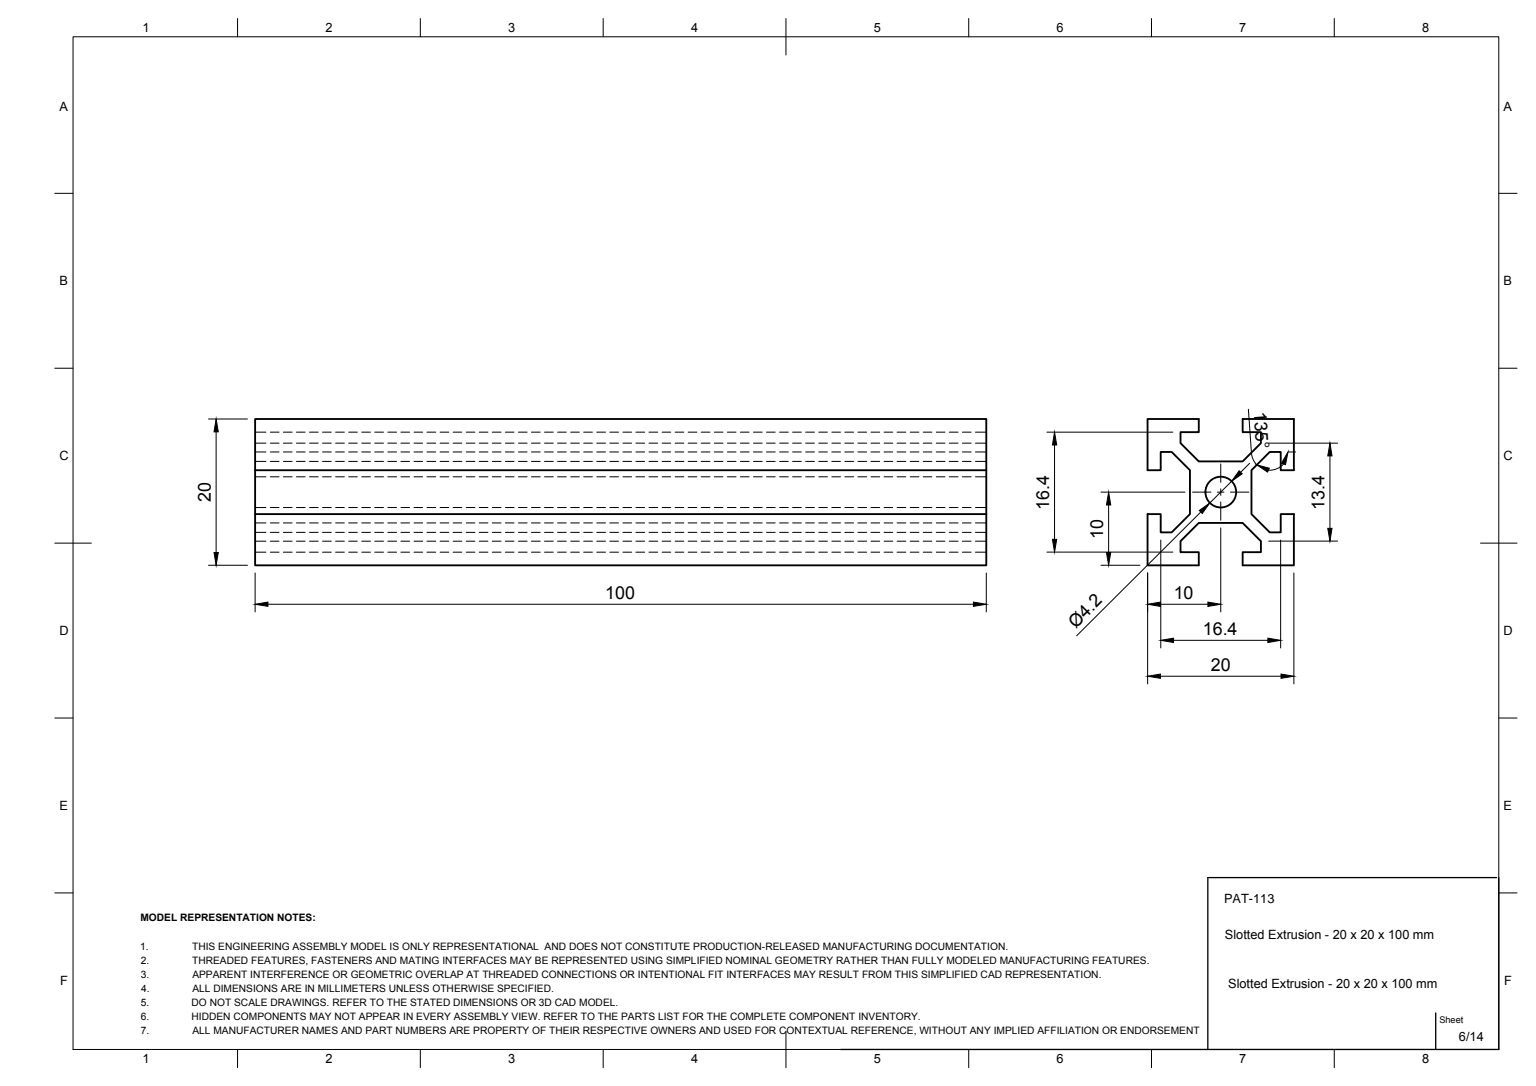
ISO-10303-21;
HEADER;
/* Generated by software containing ST-Developer
 * from STEP Tools, Inc. (www.steptools.com) 
 */

FILE_DESCRIPTION(
/* description */ ('Two-link friction support arm'),
/* implementation_level */ '2;1');

FILE_NAME(
/* name */ 'Slotted Extrusion - 20 x 20 x 100 mm.step',
/* time_stamp */ '2026-10-27T20:01:49-07:00',
/* author */ (''),
/* organization */ (''),
/* preprocessor_version */ 'ST-DEVELOPER v20.2',
/* originating_system */ 'Autodesk Translation Framework v15.17.0.0',
/* authorisation */ '');

FILE_SCHEMA (('AUTOMOTIVE_DESIGN { 1 0 10303 214 3 1 1 }'));
ENDSEC;

DATA;
#10=MECHANICAL_DESIGN_GEOMETRIC_PRESENTATION_REPRESENTATION('',(#196),#5492);
#174=SHAPE_REPRESENTATION_RELATIONSHIP('SRR','None',#5565,#185);
#185=ADVANCED_BREP_SHAPE_REPRESENTATION('',(#207),#5479);
#196=STYLED_ITEM('',(#5715),#207);
#207=MANIFOLD_SOLID_BREP('Body1',#3172);
#222=FACE_BOUND('',#605,.T.);
#223=FACE_BOUND('',#607,.T.);
#260=PLANE('',#3328);
#261=PLANE('',#3329);
#262=PLANE('',#3330);
#263=PLANE('',#3331);
#264=PLANE('',#3332);
#265=PLANE('',#3333);
#266=PLANE('',#3334);
#267=PLANE('',#3335);
#268=PLANE('',#3336);
#269=PLANE('',#3337);
#270=PLANE('',#3338);
#271=PLANE('',#3339);
#272=PLANE('',#3340);
#273=PLANE('',#3341);
#274=PLANE('',#3342);
#275=PLANE('',#3343);
#276=PLANE('',#3344);
#277=PLANE('',#3345);
#278=PLANE('',#3346);
#279=PLANE('',#3347);
#280=PLANE('',#3348);
#281=PLANE('',#3349);
#282=PLANE('',#3350);
#283=PLANE('',#3351);
#284=PLANE('',#3352);
#285=PLANE('',#3353);
#286=PLANE('',#3354);
#287=PLANE('',#3355);
#288=PLANE('',#3356);
#289=PLANE('',#3357);
#290=PLANE('',#3358);
#291=PLANE('',#3359);
#292=PLANE('',#3360);
#293=PLANE('',#3361);
#294=PLANE('',#3362);
#295=PLANE('',#3363);
#296=PLANE('',#3367);
#297=PLANE('',#3368);
#298=PLANE('',#3369);
#299=PLANE('',#3370);
#300=PLANE('',#3371);
#301=PLANE('',#3372);
#302=PLANE('',#3373);
#303=PLANE('',#3374);
#304=PLANE('',#3375);
#305=PLANE('',#3376);
#386=FACE_OUTER_BOUND('',#559,.T.);
#387=FACE_OUTER_BOUND('',#560,.T.);
#388=FACE_OUTER_BOUND('',#561,.T.);
#389=FACE_OUTER_BOUND('',#562,.T.);
#390=FACE_OUTER_BOUND('',#563,.T.);
#391=FACE_OUTER_BOUND('',#564,.T.);
#392=FACE_OUTER_BOUND('',#565,.T.);
#393=FACE_OUTER_BOUND('',#566,.T.);
#394=FACE_OUTER_BOUND('',#567,.T.);
#395=FACE_OUTER_BOUND('',#568,.T.);
#396=FACE_OUTER_BOUND('',#569,.T.);
#397=FACE_OUTER_BOUND('',#570,.T.);
#398=FACE_OUTER_BOUND('',#571,.T.);
#399=FACE_OUTER_BOUND('',#572,.T.);
#400=FACE_OUTER_BOUND('',#573,.T.);
#401=FACE_OUTER_BOUND('',#574,.T.);
#402=FACE_OUTER_BOUND('',#575,.T.);
#403=FACE_OUTER_BOUND('',#576,.T.);
#404=FACE_OUTER_BOUND('',#577,.T.);
#405=FACE_OUTER_BOUND('',#578,.T.);
#406=FACE_OUTER_BOUND('',#579,.T.);
#407=FACE_OUTER_BOUND('',#580,.T.);
#408=FACE_OUTER_BOUND('',#581,.T.);
#409=FACE_OUTER_BOUND('',#582,.T.);
#410=FACE_OUTER_BOUND('',#583,.T.);
#411=FACE_OUTER_BOUND('',#584,.T.);
#412=FACE_OUTER_BOUND('',#585,.T.);
#413=FACE_OUTER_BOUND('',#586,.T.);
#414=FACE_OUTER_BOUND('',#587,.T.);
#415=FACE_OUTER_BOUND('',#588,.T.);
#416=FACE_OUTER_BOUND('',#589,.T.);
#417=FACE_OUTER_BOUND('',#590,.T.);
#418=FACE_OUTER_BOUND('',#591,.T.);
#419=FACE_OUTER_BOUND('',#592,.T.);
#420=FACE_OUTER_BOUND('',#593,.T.);
#421=FACE_OUTER_BOUND('',#594,.T.);
#422=FACE_OUTER_BOUND('',#595,.T.);
#423=FACE_OUTER_BOUND('',#596,.T.);
#424=FACE_OUTER_BOUND('',#597,.T.);
#425=FACE_OUTER_BOUND('',#598,.T.);
#426=FACE_OUTER_BOUND('',#599,.T.);
#427=FACE_OUTER_BOUND('',#600,.T.);
#428=FACE_OUTER_BOUND('',#601,.T.);
#429=FACE_OUTER_BOUND('',#602,.T.);
#430=FACE_OUTER_BOUND('',#603,.T.);
#431=FACE_OUTER_BOUND('',#604,.T.);
#432=FACE_OUTER_BOUND('',#606,.T.);
#559=EDGE_LOOP('',(#2204,#2205,#2206,#2207));
#560=EDGE_LOOP('',(#2208,#2209,#2210,#2211));
#561=EDGE_LOOP('',(#2212,#2213,#2214,#2215));
#562=EDGE_LOOP('',(#2216,#2217,#2218,#2219));
#563=EDGE_LOOP('',(#2220,#2221,#2222,#2223));
#564=EDGE_LOOP('',(#2224,#2225,#2226,#2227));
#565=EDGE_LOOP('',(#2228,#2229,#2230,#2231));
#566=EDGE_LOOP('',(#2232,#2233,#2234,#2235));
#567=EDGE_LOOP('',(#2236,#2237,#2238,#2239));
#568=EDGE_LOOP('',(#2240,#2241,#2242,#2243));
#569=EDGE_LOOP('',(#2244,#2245,#2246,#2247));
#570=EDGE_LOOP('',(#2248,#2249,#2250,#2251));
#571=EDGE_LOOP('',(#2252,#2253,#2254,#2255));
#572=EDGE_LOOP('',(#2256,#2257,#2258,#2259));
#573=EDGE_LOOP('',(#2260,#2261,#2262,#2263));
#574=EDGE_LOOP('',(#2264,#2265,#2266,#2267));
#575=EDGE_LOOP('',(#2268,#2269,#2270,#2271));
#576=EDGE_LOOP('',(#2272,#2273,#2274,#2275));
#577=EDGE_LOOP('',(#2276,#2277,#2278,#2279));
#578=EDGE_LOOP('',(#2280,#2281,#2282,#2283));
#579=EDGE_LOOP('',(#2284,#2285,#2286,#2287));
#580=EDGE_LOOP('',(#2288,#2289,#2290,#2291));
#581=EDGE_LOOP('',(#2292,#2293,#2294,#2295));
#582=EDGE_LOOP('',(#2296,#2297,#2298,#2299));
#583=EDGE_LOOP('',(#2300,#2301,#2302,#2303));
#584=EDGE_LOOP('',(#2304,#2305,#2306,#2307));
#585=EDGE_LOOP('',(#2308,#2309,#2310,#2311));
#586=EDGE_LOOP('',(#2312,#2313,#2314,#2315));
#587=EDGE_LOOP('',(#2316,#2317,#2318,#2319));
#588=EDGE_LOOP('',(#2320,#2321,#2322,#2323));
#589=EDGE_LOOP('',(#2324,#2325,#2326,#2327));
#590=EDGE_LOOP('',(#2328,#2329,#2330,#2331));
#591=EDGE_LOOP('',(#2332,#2333,#2334,#2335));
#592=EDGE_LOOP('',(#2336,#2337,#2338,#2339));
#593=EDGE_LOOP('',(#2340,#2341,#2342,#2343));
#594=EDGE_LOOP('',(#2344,#2345,#2346,#2347));
#595=EDGE_LOOP('',(#2348,#2349,#2350,#2351));
#596=EDGE_LOOP('',(#2352,#2353,#2354,#2355));
#597=EDGE_LOOP('',(#2356,#2357,#2358,#2359));
#598=EDGE_LOOP('',(#2360,#2361,#2362,#2363));
#599=EDGE_LOOP('',(#2364,#2365,#2366,#2367));
#600=EDGE_LOOP('',(#2368,#2369,#2370,#2371));
#601=EDGE_LOOP('',(#2372,#2373,#2374,#2375));
#602=EDGE_LOOP('',(#2376,#2377,#2378,#2379));
#603=EDGE_LOOP('',(#2380,#2381,#2382,#2383));
#604=EDGE_LOOP('',(#2384,#2385,#2386,#2387,#2388,#2389,#2390,#2391,#2392,
#2393,#2394,#2395,#2396,#2397,#2398,#2399,#2400,#2401,#2402,#2403,#2404,
#2405,#2406,#2407,#2408,#2409,#2410,#2411,#2412,#2413,#2414,#2415,#2416,
#2417,#2418,#2419,#2420,#2421,#2422,#2423,#2424,#2425,#2426,#2427));
#605=EDGE_LOOP('',(#2428));
#606=EDGE_LOOP('',(#2429,#2430,#2431,#2432,#2433,#2434,#2435,#2436,#2437,
#2438,#2439,#2440,#2441,#2442,#2443,#2444,#2445,#2446,#2447,#2448,#2449,
#2450,#2451,#2452,#2453,#2454,#2455,#2456,#2457,#2458,#2459,#2460,#2461,
#2462,#2463,#2464,#2465,#2466,#2467,#2468,#2469,#2470,#2471,#2472));
#607=EDGE_LOOP('',(#2473));
#768=LINE('',#4593,#1081);
#769=LINE('',#4595,#1082);
#770=LINE('',#4597,#1083);
#771=LINE('',#4598,#1084);
#772=LINE('',#4601,#1085);
#773=LINE('',#4603,#1086);
#774=LINE('',#4604,#1087);
#775=LINE('',#4607,#1088);
#776=LINE('',#4609,#1089);
#777=LINE('',#4610,#1090);
#778=LINE('',#4613,#1091);
#779=LINE('',#4615,#1092);
#780=LINE('',#4616,#1093);
#781=LINE('',#4619,#1094);
#782=LINE('',#4621,#1095);
#783=LINE('',#4622,#1096);
#784=LINE('',#4625,#1097);
#785=LINE('',#4627,#1098);
#786=LINE('',#4628,#1099);
#787=LINE('',#4631,#1100);
#788=LINE('',#4633,#1101);
#789=LINE('',#4634,#1102);
#790=LINE('',#4637,#1103);
#791=LINE('',#4639,#1104);
#792=LINE('',#4640,#1105);
#793=LINE('',#4643,#1106);
#794=LINE('',#4645,#1107);
#795=LINE('',#4646,#1108);
#796=LINE('',#4650,#1109);
#797=LINE('',#4652,#1110);
#798=LINE('',#4654,#1111);
#799=LINE('',#4655,#1112);
#800=LINE('',#4658,#1113);
#801=LINE('',#4660,#1114);
#802=LINE('',#4661,#1115);
#803=LINE('',#4664,#1116);
#804=LINE('',#4666,#1117);
#805=LINE('',#4667,#1118);
#806=LINE('',#4670,#1119);
#807=LINE('',#4672,#1120);
#808=LINE('',#4673,#1121);
#809=LINE('',#4676,#1122);
#810=LINE('',#4678,#1123);
#811=LINE('',#4679,#1124);
#812=LINE('',#4682,#1125);
#813=LINE('',#4684,#1126);
#814=LINE('',#4685,#1127);
#815=LINE('',#4688,#1128);
#816=LINE('',#4690,#1129);
#817=LINE('',#4691,#1130);
#818=LINE('',#4694,#1131);
#819=LINE('',#4696,#1132);
#820=LINE('',#4697,#1133);
#821=LINE('',#4700,#1134);
#822=LINE('',#4702,#1135);
#823=LINE('',#4703,#1136);
#824=LINE('',#4707,#1137);
#825=LINE('',#4709,#1138);
#826=LINE('',#4711,#1139);
#827=LINE('',#4712,#1140);
#828=LINE('',#4715,#1141);
#829=LINE('',#4717,#1142);
#830=LINE('',#4718,#1143);
#831=LINE('',#4721,#1144);
#832=LINE('',#4723,#1145);
#833=LINE('',#4724,#1146);
#834=LINE('',#4727,#1147);
#835=LINE('',#4729,#1148);
#836=LINE('',#4730,#1149);
#837=LINE('',#4733,#1150);
#838=LINE('',#4735,#1151);
#839=LINE('',#4736,#1152);
#840=LINE('',#4739,#1153);
#841=LINE('',#4741,#1154);
#842=LINE('',#4742,#1155);
#843=LINE('',#4745,#1156);
#844=LINE('',#4747,#1157);
#845=LINE('',#4748,#1158);
#846=LINE('',#4751,#1159);
#847=LINE('',#4753,#1160);
#848=LINE('',#4754,#1161);
#849=LINE('',#4757,#1162);
#850=LINE('',#4759,#1163);
#851=LINE('',#4760,#1164);
#852=LINE('',#4764,#1165);
#853=LINE('',#4766,#1166);
#854=LINE('',#4768,#1167);
#855=LINE('',#4769,#1168);
#856=LINE('',#4772,#1169);
#857=LINE('',#4774,#1170);
#858=LINE('',#4775,#1171);
#859=LINE('',#4778,#1172);
#860=LINE('',#4780,#1173);
#861=LINE('',#4781,#1174);
#862=LINE('',#4784,#1175);
#863=LINE('',#4786,#1176);
#864=LINE('',#4787,#1177);
#865=LINE('',#4790,#1178);
#866=LINE('',#4792,#1179);
#867=LINE('',#4793,#1180);
#868=LINE('',#4796,#1181);
#869=LINE('',#4798,#1182);
#870=LINE('',#4799,#1183);
#871=LINE('',#4802,#1184);
#872=LINE('',#4804,#1185);
#873=LINE('',#4805,#1186);
#874=LINE('',#4808,#1187);
#875=LINE('',#4810,#1188);
#876=LINE('',#4811,#1189);
#877=LINE('',#4814,#1190);
#878=LINE('',#4816,#1191);
#879=LINE('',#4817,#1192);
#880=LINE('',#4822,#1193);
#881=LINE('',#4826,#1194);
#882=LINE('',#4828,#1195);
#883=LINE('',#4829,#1196);
#884=LINE('',#4832,#1197);
#885=LINE('',#4834,#1198);
#886=LINE('',#4835,#1199);
#887=LINE('',#4837,#1200);
#888=LINE('',#4838,#1201);
#889=LINE('',#4841,#1202);
#890=LINE('',#4843,#1203);
#891=LINE('',#4844,#1204);
#892=LINE('',#4846,#1205);
#893=LINE('',#4847,#1206);
#894=LINE('',#4850,#1207);
#895=LINE('',#4852,#1208);
#896=LINE('',#4853,#1209);
#897=LINE('',#4855,#1210);
#898=LINE('',#4856,#1211);
#899=LINE('',#4858,#1212);
#900=LINE('',#4859,#1213);
#1081=VECTOR('',#3680,1.);
#1082=VECTOR('',#3681,1.);
#1083=VECTOR('',#3682,1.);
#1084=VECTOR('',#3683,1.);
#1085=VECTOR('',#3686,1.);
#1086=VECTOR('',#3687,1.);
#1087=VECTOR('',#3688,1.);
#1088=VECTOR('',#3691,1.);
#1089=VECTOR('',#3692,1.);
#1090=VECTOR('',#3693,1.);
#1091=VECTOR('',#3696,1.);
#1092=VECTOR('',#3697,1.);
#1093=VECTOR('',#3698,1.);
#1094=VECTOR('',#3701,1.);
#1095=VECTOR('',#3702,1.);
#1096=VECTOR('',#3703,1.);
#1097=VECTOR('',#3706,1.);
#1098=VECTOR('',#3707,1.);
#1099=VECTOR('',#3708,1.);
#1100=VECTOR('',#3711,1.);
#1101=VECTOR('',#3712,1.);
#1102=VECTOR('',#3713,1.);
#1103=VECTOR('',#3716,1.);
#1104=VECTOR('',#3717,1.);
#1105=VECTOR('',#3718,1.);
#1106=VECTOR('',#3721,1.);
#1107=VECTOR('',#3722,1.);
#1108=VECTOR('',#3723,1.);
#1109=VECTOR('',#3726,1.);
#1110=VECTOR('',#3727,1.);
#1111=VECTOR('',#3728,1.);
#1112=VECTOR('',#3729,1.);
#1113=VECTOR('',#3732,1.);
#1114=VECTOR('',#3733,1.);
#1115=VECTOR('',#3734,1.);
#1116=VECTOR('',#3737,1.);
#1117=VECTOR('',#3738,1.);
#1118=VECTOR('',#3739,1.);
#1119=VECTOR('',#3742,1.);
#1120=VECTOR('',#3743,1.);
#1121=VECTOR('',#3744,1.);
#1122=VECTOR('',#3747,1.);
#1123=VECTOR('',#3748,1.);
#1124=VECTOR('',#3749,1.);
#1125=VECTOR('',#3752,1.);
#1126=VECTOR('',#3753,1.);
#1127=VECTOR('',#3754,1.);
#1128=VECTOR('',#3757,1.);
#1129=VECTOR('',#3758,1.);
#1130=VECTOR('',#3759,1.);
#1131=VECTOR('',#3762,1.);
#1132=VECTOR('',#3763,1.);
#1133=VECTOR('',#3764,1.);
#1134=VECTOR('',#3767,1.);
#1135=VECTOR('',#3768,1.);
#1136=VECTOR('',#3769,1.);
#1137=VECTOR('',#3772,1.);
#1138=VECTOR('',#3773,1.);
#1139=VECTOR('',#3774,1.);
#1140=VECTOR('',#3775,1.);
#1141=VECTOR('',#3778,1.);
#1142=VECTOR('',#3779,1.);
#1143=VECTOR('',#3780,1.);
#1144=VECTOR('',#3783,1.);
#1145=VECTOR('',#3784,1.);
#1146=VECTOR('',#3785,1.);
#1147=VECTOR('',#3788,1.);
#1148=VECTOR('',#3789,1.);
#1149=VECTOR('',#3790,1.);
#1150=VECTOR('',#3793,1.);
#1151=VECTOR('',#3794,1.);
#1152=VECTOR('',#3795,1.);
#1153=VECTOR('',#3798,1.);
#1154=VECTOR('',#3799,1.);
#1155=VECTOR('',#3800,1.);
#1156=VECTOR('',#3803,1.);
#1157=VECTOR('',#3804,1.);
#1158=VECTOR('',#3805,1.);
#1159=VECTOR('',#3808,1.);
#1160=VECTOR('',#3809,1.);
#1161=VECTOR('',#3810,1.);
#1162=VECTOR('',#3813,1.);
#1163=VECTOR('',#3814,1.);
#1164=VECTOR('',#3815,1.);
#1165=VECTOR('',#3818,1.);
#1166=VECTOR('',#3819,1.);
#1167=VECTOR('',#3820,1.);
#1168=VECTOR('',#3821,1.);
#1169=VECTOR('',#3824,1.);
#1170=VECTOR('',#3825,1.);
#1171=VECTOR('',#3826,1.);
#1172=VECTOR('',#3829,1.);
#1173=VECTOR('',#3830,1.);
#1174=VECTOR('',#3831,1.);
#1175=VECTOR('',#3834,1.);
#1176=VECTOR('',#3835,1.);
#1177=VECTOR('',#3836,1.);
#1178=VECTOR('',#3839,1.);
#1179=VECTOR('',#3840,1.);
#1180=VECTOR('',#3841,1.);
#1181=VECTOR('',#3844,1.);
#1182=VECTOR('',#3845,1.);
#1183=VECTOR('',#3846,1.);
#1184=VECTOR('',#3849,1.);
#1185=VECTOR('',#3850,1.);
#1186=VECTOR('',#3851,1.);
#1187=VECTOR('',#3854,1.);
#1188=VECTOR('',#3855,1.);
#1189=VECTOR('',#3856,1.);
#1190=VECTOR('',#3859,1.);
#1191=VECTOR('',#3860,1.);
#1192=VECTOR('',#3861,1.);
#1193=VECTOR('',#3866,0.21);
#1194=VECTOR('',#3871,1.);
#1195=VECTOR('',#3872,1.);
#1196=VECTOR('',#3873,1.);
#1197=VECTOR('',#3876,1.);
#1198=VECTOR('',#3877,1.);
#1199=VECTOR('',#3878,1.);
#1200=VECTOR('',#3881,1.);
#1201=VECTOR('',#3882,1.);
#1202=VECTOR('',#3885,1.);
#1203=VECTOR('',#3886,1.);
#1204=VECTOR('',#3887,1.);
#1205=VECTOR('',#3890,1.);
#1206=VECTOR('',#3891,1.);
#1207=VECTOR('',#3894,1.);
#1208=VECTOR('',#3895,1.);
#1209=VECTOR('',#3896,1.);
#1210=VECTOR('',#3899,1.);
#1211=VECTOR('',#3900,1.);
#1212=VECTOR('',#3903,1.);
#1213=VECTOR('',#3904,1.);
#1373=CIRCLE('',#3365,0.21);
#1374=CIRCLE('',#3366,0.21);
#1471=VERTEX_POINT('',#4591);
#1472=VERTEX_POINT('',#4592);
#1473=VERTEX_POINT('',#4594);
#1474=VERTEX_POINT('',#4596);
#1475=VERTEX_POINT('',#4600);
#1476=VERTEX_POINT('',#4602);
#1477=VERTEX_POINT('',#4606);
#1478=VERTEX_POINT('',#4608);
#1479=VERTEX_POINT('',#4612);
#1480=VERTEX_POINT('',#4614);
#1481=VERTEX_POINT('',#4618);
#1482=VERTEX_POINT('',#4620);
#1483=VERTEX_POINT('',#4624);
#1484=VERTEX_POINT('',#4626);
#1485=VERTEX_POINT('',#4630);
#1486=VERTEX_POINT('',#4632);
#1487=VERTEX_POINT('',#4636);
#1488=VERTEX_POINT('',#4638);
#1489=VERTEX_POINT('',#4642);
#1490=VERTEX_POINT('',#4644);
#1491=VERTEX_POINT('',#4648);
#1492=VERTEX_POINT('',#4649);
#1493=VERTEX_POINT('',#4651);
#1494=VERTEX_POINT('',#4653);
#1495=VERTEX_POINT('',#4657);
#1496=VERTEX_POINT('',#4659);
#1497=VERTEX_POINT('',#4663);
#1498=VERTEX_POINT('',#4665);
#1499=VERTEX_POINT('',#4669);
#1500=VERTEX_POINT('',#4671);
#1501=VERTEX_POINT('',#4675);
#1502=VERTEX_POINT('',#4677);
#1503=VERTEX_POINT('',#4681);
#1504=VERTEX_POINT('',#4683);
#1505=VERTEX_POINT('',#4687);
#1506=VERTEX_POINT('',#4689);
#1507=VERTEX_POINT('',#4693);
#1508=VERTEX_POINT('',#4695);
#1509=VERTEX_POINT('',#4699);
#1510=VERTEX_POINT('',#4701);
#1511=VERTEX_POINT('',#4705);
#1512=VERTEX_POINT('',#4706);
#1513=VERTEX_POINT('',#4708);
#1514=VERTEX_POINT('',#4710);
#1515=VERTEX_POINT('',#4714);
#1516=VERTEX_POINT('',#4716);
#1517=VERTEX_POINT('',#4720);
#1518=VERTEX_POINT('',#4722);
#1519=VERTEX_POINT('',#4726);
#1520=VERTEX_POINT('',#4728);
#1521=VERTEX_POINT('',#4732);
#1522=VERTEX_POINT('',#4734);
#1523=VERTEX_POINT('',#4738);
#1524=VERTEX_POINT('',#4740);
#1525=VERTEX_POINT('',#4744);
#1526=VERTEX_POINT('',#4746);
#1527=VERTEX_POINT('',#4750);
#1528=VERTEX_POINT('',#4752);
#1529=VERTEX_POINT('',#4756);
#1530=VERTEX_POINT('',#4758);
#1531=VERTEX_POINT('',#4762);
#1532=VERTEX_POINT('',#4763);
#1533=VERTEX_POINT('',#4765);
#1534=VERTEX_POINT('',#4767);
#1535=VERTEX_POINT('',#4771);
#1536=VERTEX_POINT('',#4773);
#1537=VERTEX_POINT('',#4777);
#1538=VERTEX_POINT('',#4779);
#1539=VERTEX_POINT('',#4783);
#1540=VERTEX_POINT('',#4785);
#1541=VERTEX_POINT('',#4789);
#1542=VERTEX_POINT('',#4791);
#1543=VERTEX_POINT('',#4795);
#1544=VERTEX_POINT('',#4797);
#1545=VERTEX_POINT('',#4801);
#1546=VERTEX_POINT('',#4803);
#1547=VERTEX_POINT('',#4807);
#1548=VERTEX_POINT('',#4809);
#1549=VERTEX_POINT('',#4813);
#1550=VERTEX_POINT('',#4815);
#1551=VERTEX_POINT('',#4819);
#1552=VERTEX_POINT('',#4821);
#1553=VERTEX_POINT('',#4825);
#1554=VERTEX_POINT('',#4827);
#1555=VERTEX_POINT('',#4831);
#1556=VERTEX_POINT('',#4833);
#1557=VERTEX_POINT('',#4840);
#1558=VERTEX_POINT('',#4842);
#1559=VERTEX_POINT('',#4849);
#1560=VERTEX_POINT('',#4851);
#1756=EDGE_CURVE('',#1471,#1472,#768,.T.);
#1757=EDGE_CURVE('',#1471,#1473,#769,.T.);
#1758=EDGE_CURVE('',#1474,#1473,#770,.T.);
#1759=EDGE_CURVE('',#1472,#1474,#771,.T.);
#1760=EDGE_CURVE('',#1475,#1471,#772,.T.);
#1761=EDGE_CURVE('',#1475,#1476,#773,.T.);
#1762=EDGE_CURVE('',#1473,#1476,#774,.T.);
#1763=EDGE_CURVE('',#1477,#1475,#775,.T.);
#1764=EDGE_CURVE('',#1477,#1478,#776,.T.);
#1765=EDGE_CURVE('',#1476,#1478,#777,.T.);
#1766=EDGE_CURVE('',#1479,#1477,#778,.T.);
#1767=EDGE_CURVE('',#1479,#1480,#779,.T.);
#1768=EDGE_CURVE('',#1478,#1480,#780,.T.);
#1769=EDGE_CURVE('',#1481,#1479,#781,.T.);
#1770=EDGE_CURVE('',#1481,#1482,#782,.T.);
#1771=EDGE_CURVE('',#1480,#1482,#783,.T.);
#1772=EDGE_CURVE('',#1483,#1481,#784,.T.);
#1773=EDGE_CURVE('',#1483,#1484,#785,.T.);
#1774=EDGE_CURVE('',#1482,#1484,#786,.T.);
#1775=EDGE_CURVE('',#1485,#1483,#787,.T.);
#1776=EDGE_CURVE('',#1485,#1486,#788,.T.);
#1777=EDGE_CURVE('',#1484,#1486,#789,.T.);
#1778=EDGE_CURVE('',#1487,#1485,#790,.T.);
#1779=EDGE_CURVE('',#1487,#1488,#791,.T.);
#1780=EDGE_CURVE('',#1486,#1488,#792,.T.);
#1781=EDGE_CURVE('',#1489,#1487,#793,.T.);
#1782=EDGE_CURVE('',#1490,#1489,#794,.T.);
#1783=EDGE_CURVE('',#1488,#1490,#795,.T.);
#1784=EDGE_CURVE('',#1491,#1492,#796,.T.);
#1785=EDGE_CURVE('',#1491,#1493,#797,.T.);
#1786=EDGE_CURVE('',#1494,#1493,#798,.T.);
#1787=EDGE_CURVE('',#1492,#1494,#799,.T.);
#1788=EDGE_CURVE('',#1495,#1491,#800,.T.);
#1789=EDGE_CURVE('',#1495,#1496,#801,.T.);
#1790=EDGE_CURVE('',#1493,#1496,#802,.T.);
#1791=EDGE_CURVE('',#1497,#1495,#803,.T.);
#1792=EDGE_CURVE('',#1497,#1498,#804,.T.);
#1793=EDGE_CURVE('',#1496,#1498,#805,.T.);
#1794=EDGE_CURVE('',#1499,#1497,#806,.T.);
#1795=EDGE_CURVE('',#1499,#1500,#807,.T.);
#1796=EDGE_CURVE('',#1498,#1500,#808,.T.);
#1797=EDGE_CURVE('',#1501,#1499,#809,.T.);
#1798=EDGE_CURVE('',#1501,#1502,#810,.T.);
#1799=EDGE_CURVE('',#1500,#1502,#811,.T.);
#1800=EDGE_CURVE('',#1503,#1501,#812,.T.);
#1801=EDGE_CURVE('',#1503,#1504,#813,.T.);
#1802=EDGE_CURVE('',#1502,#1504,#814,.T.);
#1803=EDGE_CURVE('',#1505,#1503,#815,.T.);
#1804=EDGE_CURVE('',#1505,#1506,#816,.T.);
#1805=EDGE_CURVE('',#1504,#1506,#817,.T.);
#1806=EDGE_CURVE('',#1507,#1505,#818,.T.);
#1807=EDGE_CURVE('',#1507,#1508,#819,.T.);
#1808=EDGE_CURVE('',#1506,#1508,#820,.T.);
#1809=EDGE_CURVE('',#1509,#1507,#821,.T.);
#1810=EDGE_CURVE('',#1510,#1509,#822,.T.);
#1811=EDGE_CURVE('',#1508,#1510,#823,.T.);
#1812=EDGE_CURVE('',#1511,#1512,#824,.T.);
#1813=EDGE_CURVE('',#1511,#1513,#825,.T.);
#1814=EDGE_CURVE('',#1514,#1513,#826,.T.);
#1815=EDGE_CURVE('',#1512,#1514,#827,.T.);
#1816=EDGE_CURVE('',#1515,#1511,#828,.T.);
#1817=EDGE_CURVE('',#1515,#1516,#829,.T.);
#1818=EDGE_CURVE('',#1513,#1516,#830,.T.);
#1819=EDGE_CURVE('',#1517,#1515,#831,.T.);
#1820=EDGE_CURVE('',#1517,#1518,#832,.T.);
#1821=EDGE_CURVE('',#1516,#1518,#833,.T.);
#1822=EDGE_CURVE('',#1519,#1517,#834,.T.);
#1823=EDGE_CURVE('',#1519,#1520,#835,.T.);
#1824=EDGE_CURVE('',#1518,#1520,#836,.T.);
#1825=EDGE_CURVE('',#1521,#1519,#837,.T.);
#1826=EDGE_CURVE('',#1521,#1522,#838,.T.);
#1827=EDGE_CURVE('',#1520,#1522,#839,.T.);
#1828=EDGE_CURVE('',#1523,#1521,#840,.T.);
#1829=EDGE_CURVE('',#1523,#1524,#841,.T.);
#1830=EDGE_CURVE('',#1522,#1524,#842,.T.);
#1831=EDGE_CURVE('',#1525,#1523,#843,.T.);
#1832=EDGE_CURVE('',#1525,#1526,#844,.T.);
#1833=EDGE_CURVE('',#1524,#1526,#845,.T.);
#1834=EDGE_CURVE('',#1527,#1525,#846,.T.);
#1835=EDGE_CURVE('',#1527,#1528,#847,.T.);
#1836=EDGE_CURVE('',#1526,#1528,#848,.T.);
#1837=EDGE_CURVE('',#1529,#1527,#849,.T.);
#1838=EDGE_CURVE('',#1530,#1529,#850,.T.);
#1839=EDGE_CURVE('',#1528,#1530,#851,.T.);
#1840=EDGE_CURVE('',#1531,#1532,#852,.T.);
#1841=EDGE_CURVE('',#1531,#1533,#853,.T.);
#1842=EDGE_CURVE('',#1534,#1533,#854,.T.);
#1843=EDGE_CURVE('',#1532,#1534,#855,.T.);
#1844=EDGE_CURVE('',#1535,#1531,#856,.T.);
#1845=EDGE_CURVE('',#1535,#1536,#857,.T.);
#1846=EDGE_CURVE('',#1533,#1536,#858,.T.);
#1847=EDGE_CURVE('',#1537,#1535,#859,.T.);
#1848=EDGE_CURVE('',#1537,#1538,#860,.T.);
#1849=EDGE_CURVE('',#1536,#1538,#861,.T.);
#1850=EDGE_CURVE('',#1539,#1537,#862,.T.);
#1851=EDGE_CURVE('',#1539,#1540,#863,.T.);
#1852=EDGE_CURVE('',#1538,#1540,#864,.T.);
#1853=EDGE_CURVE('',#1541,#1539,#865,.T.);
#1854=EDGE_CURVE('',#1541,#1542,#866,.T.);
#1855=EDGE_CURVE('',#1540,#1542,#867,.T.);
#1856=EDGE_CURVE('',#1543,#1541,#868,.T.);
#1857=EDGE_CURVE('',#1543,#1544,#869,.T.);
#1858=EDGE_CURVE('',#1542,#1544,#870,.T.);
#1859=EDGE_CURVE('',#1545,#1543,#871,.T.);
#1860=EDGE_CURVE('',#1545,#1546,#872,.T.);
#1861=EDGE_CURVE('',#1544,#1546,#873,.T.);
#1862=EDGE_CURVE('',#1547,#1545,#874,.T.);
#1863=EDGE_CURVE('',#1547,#1548,#875,.T.);
#1864=EDGE_CURVE('',#1546,#1548,#876,.T.);
#1865=EDGE_CURVE('',#1549,#1547,#877,.T.);
#1866=EDGE_CURVE('',#1550,#1549,#878,.T.);
#1867=EDGE_CURVE('',#1548,#1550,#879,.T.);
#1868=EDGE_CURVE('',#1551,#1551,#1373,.T.);
#1869=EDGE_CURVE('',#1551,#1552,#880,.T.);
#1870=EDGE_CURVE('',#1552,#1552,#1374,.T.);
#1871=EDGE_CURVE('',#1489,#1553,#881,.T.);
#1872=EDGE_CURVE('',#1553,#1554,#882,.T.);
#1873=EDGE_CURVE('',#1490,#1554,#883,.T.);
#1874=EDGE_CURVE('',#1555,#1474,#884,.T.);
#1875=EDGE_CURVE('',#1556,#1555,#885,.T.);
#1876=EDGE_CURVE('',#1556,#1472,#886,.T.);
#1877=EDGE_CURVE('',#1509,#1556,#887,.T.);
#1878=EDGE_CURVE('',#1510,#1555,#888,.T.);
#1879=EDGE_CURVE('',#1557,#1494,#889,.T.);
#1880=EDGE_CURVE('',#1558,#1557,#890,.T.);
#1881=EDGE_CURVE('',#1558,#1492,#891,.T.);
#1882=EDGE_CURVE('',#1529,#1558,#892,.T.);
#1883=EDGE_CURVE('',#1530,#1557,#893,.T.);
#1884=EDGE_CURVE('',#1559,#1514,#894,.T.);
#1885=EDGE_CURVE('',#1560,#1559,#895,.T.);
#1886=EDGE_CURVE('',#1560,#1512,#896,.T.);
#1887=EDGE_CURVE('',#1549,#1560,#897,.T.);
#1888=EDGE_CURVE('',#1550,#1559,#898,.T.);
#1889=EDGE_CURVE('',#1554,#1534,#899,.T.);
#1890=EDGE_CURVE('',#1553,#1532,#900,.T.);
#2204=ORIENTED_EDGE('',*,*,#1756,.F.);
#2205=ORIENTED_EDGE('',*,*,#1757,.T.);
#2206=ORIENTED_EDGE('',*,*,#1758,.F.);
#2207=ORIENTED_EDGE('',*,*,#1759,.F.);
#2208=ORIENTED_EDGE('',*,*,#1760,.F.);
#2209=ORIENTED_EDGE('',*,*,#1761,.T.);
#2210=ORIENTED_EDGE('',*,*,#1762,.F.);
#2211=ORIENTED_EDGE('',*,*,#1757,.F.);
#2212=ORIENTED_EDGE('',*,*,#1763,.F.);
#2213=ORIENTED_EDGE('',*,*,#1764,.T.);
#2214=ORIENTED_EDGE('',*,*,#1765,.F.);
#2215=ORIENTED_EDGE('',*,*,#1761,.F.);
#2216=ORIENTED_EDGE('',*,*,#1766,.F.);
#2217=ORIENTED_EDGE('',*,*,#1767,.T.);
#2218=ORIENTED_EDGE('',*,*,#1768,.F.);
#2219=ORIENTED_EDGE('',*,*,#1764,.F.);
#2220=ORIENTED_EDGE('',*,*,#1769,.F.);
#2221=ORIENTED_EDGE('',*,*,#1770,.T.);
#2222=ORIENTED_EDGE('',*,*,#1771,.F.);
#2223=ORIENTED_EDGE('',*,*,#1767,.F.);
#2224=ORIENTED_EDGE('',*,*,#1772,.F.);
#2225=ORIENTED_EDGE('',*,*,#1773,.T.);
#2226=ORIENTED_EDGE('',*,*,#1774,.F.);
#2227=ORIENTED_EDGE('',*,*,#1770,.F.);
#2228=ORIENTED_EDGE('',*,*,#1775,.F.);
#2229=ORIENTED_EDGE('',*,*,#1776,.T.);
#2230=ORIENTED_EDGE('',*,*,#1777,.F.);
#2231=ORIENTED_EDGE('',*,*,#1773,.F.);
#2232=ORIENTED_EDGE('',*,*,#1778,.F.);
#2233=ORIENTED_EDGE('',*,*,#1779,.T.);
#2234=ORIENTED_EDGE('',*,*,#1780,.F.);
#2235=ORIENTED_EDGE('',*,*,#1776,.F.);
#2236=ORIENTED_EDGE('',*,*,#1781,.F.);
#2237=ORIENTED_EDGE('',*,*,#1782,.F.);
#2238=ORIENTED_EDGE('',*,*,#1783,.F.);
#2239=ORIENTED_EDGE('',*,*,#1779,.F.);
#2240=ORIENTED_EDGE('',*,*,#1784,.F.);
#2241=ORIENTED_EDGE('',*,*,#1785,.T.);
#2242=ORIENTED_EDGE('',*,*,#1786,.F.);
#2243=ORIENTED_EDGE('',*,*,#1787,.F.);
#2244=ORIENTED_EDGE('',*,*,#1788,.F.);
#2245=ORIENTED_EDGE('',*,*,#1789,.T.);
#2246=ORIENTED_EDGE('',*,*,#1790,.F.);
#2247=ORIENTED_EDGE('',*,*,#1785,.F.);
#2248=ORIENTED_EDGE('',*,*,#1791,.F.);
#2249=ORIENTED_EDGE('',*,*,#1792,.T.);
#2250=ORIENTED_EDGE('',*,*,#1793,.F.);
#2251=ORIENTED_EDGE('',*,*,#1789,.F.);
#2252=ORIENTED_EDGE('',*,*,#1794,.F.);
#2253=ORIENTED_EDGE('',*,*,#1795,.T.);
#2254=ORIENTED_EDGE('',*,*,#1796,.F.);
#2255=ORIENTED_EDGE('',*,*,#1792,.F.);
#2256=ORIENTED_EDGE('',*,*,#1797,.F.);
#2257=ORIENTED_EDGE('',*,*,#1798,.T.);
#2258=ORIENTED_EDGE('',*,*,#1799,.F.);
#2259=ORIENTED_EDGE('',*,*,#1795,.F.);
#2260=ORIENTED_EDGE('',*,*,#1800,.F.);
#2261=ORIENTED_EDGE('',*,*,#1801,.T.);
#2262=ORIENTED_EDGE('',*,*,#1802,.F.);
#2263=ORIENTED_EDGE('',*,*,#1798,.F.);
#2264=ORIENTED_EDGE('',*,*,#1803,.F.);
#2265=ORIENTED_EDGE('',*,*,#1804,.T.);
#2266=ORIENTED_EDGE('',*,*,#1805,.F.);
#2267=ORIENTED_EDGE('',*,*,#1801,.F.);
#2268=ORIENTED_EDGE('',*,*,#1806,.F.);
#2269=ORIENTED_EDGE('',*,*,#1807,.T.);
#2270=ORIENTED_EDGE('',*,*,#1808,.F.);
#2271=ORIENTED_EDGE('',*,*,#1804,.F.);
#2272=ORIENTED_EDGE('',*,*,#1809,.F.);
#2273=ORIENTED_EDGE('',*,*,#1810,.F.);
#2274=ORIENTED_EDGE('',*,*,#1811,.F.);
#2275=ORIENTED_EDGE('',*,*,#1807,.F.);
#2276=ORIENTED_EDGE('',*,*,#1812,.F.);
#2277=ORIENTED_EDGE('',*,*,#1813,.T.);
#2278=ORIENTED_EDGE('',*,*,#1814,.F.);
#2279=ORIENTED_EDGE('',*,*,#1815,.F.);
#2280=ORIENTED_EDGE('',*,*,#1816,.F.);
#2281=ORIENTED_EDGE('',*,*,#1817,.T.);
#2282=ORIENTED_EDGE('',*,*,#1818,.F.);
#2283=ORIENTED_EDGE('',*,*,#1813,.F.);
#2284=ORIENTED_EDGE('',*,*,#1819,.F.);
#2285=ORIENTED_EDGE('',*,*,#1820,.T.);
#2286=ORIENTED_EDGE('',*,*,#1821,.F.);
#2287=ORIENTED_EDGE('',*,*,#1817,.F.);
#2288=ORIENTED_EDGE('',*,*,#1822,.F.);
#2289=ORIENTED_EDGE('',*,*,#1823,.T.);
#2290=ORIENTED_EDGE('',*,*,#1824,.F.);
#2291=ORIENTED_EDGE('',*,*,#1820,.F.);
#2292=ORIENTED_EDGE('',*,*,#1825,.F.);
#2293=ORIENTED_EDGE('',*,*,#1826,.T.);
#2294=ORIENTED_EDGE('',*,*,#1827,.F.);
#2295=ORIENTED_EDGE('',*,*,#1823,.F.);
#2296=ORIENTED_EDGE('',*,*,#1828,.F.);
#2297=ORIENTED_EDGE('',*,*,#1829,.T.);
#2298=ORIENTED_EDGE('',*,*,#1830,.F.);
#2299=ORIENTED_EDGE('',*,*,#1826,.F.);
#2300=ORIENTED_EDGE('',*,*,#1831,.F.);
#2301=ORIENTED_EDGE('',*,*,#1832,.T.);
#2302=ORIENTED_EDGE('',*,*,#1833,.F.);
#2303=ORIENTED_EDGE('',*,*,#1829,.F.);
#2304=ORIENTED_EDGE('',*,*,#1834,.F.);
#2305=ORIENTED_EDGE('',*,*,#1835,.T.);
#2306=ORIENTED_EDGE('',*,*,#1836,.F.);
#2307=ORIENTED_EDGE('',*,*,#1832,.F.);
#2308=ORIENTED_EDGE('',*,*,#1837,.F.);
#2309=ORIENTED_EDGE('',*,*,#1838,.F.);
#2310=ORIENTED_EDGE('',*,*,#1839,.F.);
#2311=ORIENTED_EDGE('',*,*,#1835,.F.);
#2312=ORIENTED_EDGE('',*,*,#1840,.F.);
#2313=ORIENTED_EDGE('',*,*,#1841,.T.);
#2314=ORIENTED_EDGE('',*,*,#1842,.F.);
#2315=ORIENTED_EDGE('',*,*,#1843,.F.);
#2316=ORIENTED_EDGE('',*,*,#1844,.F.);
#2317=ORIENTED_EDGE('',*,*,#1845,.T.);
#2318=ORIENTED_EDGE('',*,*,#1846,.F.);
#2319=ORIENTED_EDGE('',*,*,#1841,.F.);
#2320=ORIENTED_EDGE('',*,*,#1847,.F.);
#2321=ORIENTED_EDGE('',*,*,#1848,.T.);
#2322=ORIENTED_EDGE('',*,*,#1849,.F.);
#2323=ORIENTED_EDGE('',*,*,#1845,.F.);
#2324=ORIENTED_EDGE('',*,*,#1850,.F.);
#2325=ORIENTED_EDGE('',*,*,#1851,.T.);
#2326=ORIENTED_EDGE('',*,*,#1852,.F.);
#2327=ORIENTED_EDGE('',*,*,#1848,.F.);
#2328=ORIENTED_EDGE('',*,*,#1853,.F.);
#2329=ORIENTED_EDGE('',*,*,#1854,.T.);
#2330=ORIENTED_EDGE('',*,*,#1855,.F.);
#2331=ORIENTED_EDGE('',*,*,#1851,.F.);
#2332=ORIENTED_EDGE('',*,*,#1856,.F.);
#2333=ORIENTED_EDGE('',*,*,#1857,.T.);
#2334=ORIENTED_EDGE('',*,*,#1858,.F.);
#2335=ORIENTED_EDGE('',*,*,#1854,.F.);
#2336=ORIENTED_EDGE('',*,*,#1859,.F.);
#2337=ORIENTED_EDGE('',*,*,#1860,.T.);
#2338=ORIENTED_EDGE('',*,*,#1861,.F.);
#2339=ORIENTED_EDGE('',*,*,#1857,.F.);
#2340=ORIENTED_EDGE('',*,*,#1862,.F.);
#2341=ORIENTED_EDGE('',*,*,#1863,.T.);
#2342=ORIENTED_EDGE('',*,*,#1864,.F.);
#2343=ORIENTED_EDGE('',*,*,#1860,.F.);
#2344=ORIENTED_EDGE('',*,*,#1865,.F.);
#2345=ORIENTED_EDGE('',*,*,#1866,.F.);
#2346=ORIENTED_EDGE('',*,*,#1867,.F.);
#2347=ORIENTED_EDGE('',*,*,#1863,.F.);
#2348=ORIENTED_EDGE('',*,*,#1868,.F.);
#2349=ORIENTED_EDGE('',*,*,#1869,.T.);
#2350=ORIENTED_EDGE('',*,*,#1870,.F.);
#2351=ORIENTED_EDGE('',*,*,#1869,.F.);
#2352=ORIENTED_EDGE('',*,*,#1782,.T.);
#2353=ORIENTED_EDGE('',*,*,#1871,.T.);
#2354=ORIENTED_EDGE('',*,*,#1872,.T.);
#2355=ORIENTED_EDGE('',*,*,#1873,.F.);
#2356=ORIENTED_EDGE('',*,*,#1759,.T.);
#2357=ORIENTED_EDGE('',*,*,#1874,.F.);
#2358=ORIENTED_EDGE('',*,*,#1875,.F.);
#2359=ORIENTED_EDGE('',*,*,#1876,.T.);
#2360=ORIENTED_EDGE('',*,*,#1810,.T.);
#2361=ORIENTED_EDGE('',*,*,#1877,.T.);
#2362=ORIENTED_EDGE('',*,*,#1875,.T.);
#2363=ORIENTED_EDGE('',*,*,#1878,.F.);
#2364=ORIENTED_EDGE('',*,*,#1787,.T.);
#2365=ORIENTED_EDGE('',*,*,#1879,.F.);
#2366=ORIENTED_EDGE('',*,*,#1880,.F.);
#2367=ORIENTED_EDGE('',*,*,#1881,.T.);
#2368=ORIENTED_EDGE('',*,*,#1838,.T.);
#2369=ORIENTED_EDGE('',*,*,#1882,.T.);
#2370=ORIENTED_EDGE('',*,*,#1880,.T.);
#2371=ORIENTED_EDGE('',*,*,#1883,.F.);
#2372=ORIENTED_EDGE('',*,*,#1815,.T.);
#2373=ORIENTED_EDGE('',*,*,#1884,.F.);
#2374=ORIENTED_EDGE('',*,*,#1885,.F.);
#2375=ORIENTED_EDGE('',*,*,#1886,.T.);
#2376=ORIENTED_EDGE('',*,*,#1866,.T.);
#2377=ORIENTED_EDGE('',*,*,#1887,.T.);
#2378=ORIENTED_EDGE('',*,*,#1885,.T.);
#2379=ORIENTED_EDGE('',*,*,#1888,.F.);
#2380=ORIENTED_EDGE('',*,*,#1843,.T.);
#2381=ORIENTED_EDGE('',*,*,#1889,.F.);
#2382=ORIENTED_EDGE('',*,*,#1872,.F.);
#2383=ORIENTED_EDGE('',*,*,#1890,.T.);
#2384=ORIENTED_EDGE('',*,*,#1758,.T.);
#2385=ORIENTED_EDGE('',*,*,#1762,.T.);
#2386=ORIENTED_EDGE('',*,*,#1765,.T.);
#2387=ORIENTED_EDGE('',*,*,#1768,.T.);
#2388=ORIENTED_EDGE('',*,*,#1771,.T.);
#2389=ORIENTED_EDGE('',*,*,#1774,.T.);
#2390=ORIENTED_EDGE('',*,*,#1777,.T.);
#2391=ORIENTED_EDGE('',*,*,#1780,.T.);
#2392=ORIENTED_EDGE('',*,*,#1783,.T.);
#2393=ORIENTED_EDGE('',*,*,#1873,.T.);
#2394=ORIENTED_EDGE('',*,*,#1889,.T.);
#2395=ORIENTED_EDGE('',*,*,#1842,.T.);
#2396=ORIENTED_EDGE('',*,*,#1846,.T.);
#2397=ORIENTED_EDGE('',*,*,#1849,.T.);
#2398=ORIENTED_EDGE('',*,*,#1852,.T.);
#2399=ORIENTED_EDGE('',*,*,#1855,.T.);
#2400=ORIENTED_EDGE('',*,*,#1858,.T.);
#2401=ORIENTED_EDGE('',*,*,#1861,.T.);
#2402=ORIENTED_EDGE('',*,*,#1864,.T.);
#2403=ORIENTED_EDGE('',*,*,#1867,.T.);
#2404=ORIENTED_EDGE('',*,*,#1888,.T.);
#2405=ORIENTED_EDGE('',*,*,#1884,.T.);
#2406=ORIENTED_EDGE('',*,*,#1814,.T.);
#2407=ORIENTED_EDGE('',*,*,#1818,.T.);
#2408=ORIENTED_EDGE('',*,*,#1821,.T.);
#2409=ORIENTED_EDGE('',*,*,#1824,.T.);
#2410=ORIENTED_EDGE('',*,*,#1827,.T.);
#2411=ORIENTED_EDGE('',*,*,#1830,.T.);
#2412=ORIENTED_EDGE('',*,*,#1833,.T.);
#2413=ORIENTED_EDGE('',*,*,#1836,.T.);
#2414=ORIENTED_EDGE('',*,*,#1839,.T.);
#2415=ORIENTED_EDGE('',*,*,#1883,.T.);
#2416=ORIENTED_EDGE('',*,*,#1879,.T.);
#2417=ORIENTED_EDGE('',*,*,#1786,.T.);
#2418=ORIENTED_EDGE('',*,*,#1790,.T.);
#2419=ORIENTED_EDGE('',*,*,#1793,.T.);
#2420=ORIENTED_EDGE('',*,*,#1796,.T.);
#2421=ORIENTED_EDGE('',*,*,#1799,.T.);
#2422=ORIENTED_EDGE('',*,*,#1802,.T.);
#2423=ORIENTED_EDGE('',*,*,#1805,.T.);
#2424=ORIENTED_EDGE('',*,*,#1808,.T.);
#2425=ORIENTED_EDGE('',*,*,#1811,.T.);
#2426=ORIENTED_EDGE('',*,*,#1878,.T.);
#2427=ORIENTED_EDGE('',*,*,#1874,.T.);
#2428=ORIENTED_EDGE('',*,*,#1870,.T.);
#2429=ORIENTED_EDGE('',*,*,#1756,.T.);
#2430=ORIENTED_EDGE('',*,*,#1876,.F.);
#2431=ORIENTED_EDGE('',*,*,#1877,.F.);
#2432=ORIENTED_EDGE('',*,*,#1809,.T.);
#2433=ORIENTED_EDGE('',*,*,#1806,.T.);
#2434=ORIENTED_EDGE('',*,*,#1803,.T.);
#2435=ORIENTED_EDGE('',*,*,#1800,.T.);
#2436=ORIENTED_EDGE('',*,*,#1797,.T.);
#2437=ORIENTED_EDGE('',*,*,#1794,.T.);
#2438=ORIENTED_EDGE('',*,*,#1791,.T.);
#2439=ORIENTED_EDGE('',*,*,#1788,.T.);
#2440=ORIENTED_EDGE('',*,*,#1784,.T.);
#2441=ORIENTED_EDGE('',*,*,#1881,.F.);
#2442=ORIENTED_EDGE('',*,*,#1882,.F.);
#2443=ORIENTED_EDGE('',*,*,#1837,.T.);
#2444=ORIENTED_EDGE('',*,*,#1834,.T.);
#2445=ORIENTED_EDGE('',*,*,#1831,.T.);
#2446=ORIENTED_EDGE('',*,*,#1828,.T.);
#2447=ORIENTED_EDGE('',*,*,#1825,.T.);
#2448=ORIENTED_EDGE('',*,*,#1822,.T.);
#2449=ORIENTED_EDGE('',*,*,#1819,.T.);
#2450=ORIENTED_EDGE('',*,*,#1816,.T.);
#2451=ORIENTED_EDGE('',*,*,#1812,.T.);
#2452=ORIENTED_EDGE('',*,*,#1886,.F.);
#2453=ORIENTED_EDGE('',*,*,#1887,.F.);
#2454=ORIENTED_EDGE('',*,*,#1865,.T.);
#2455=ORIENTED_EDGE('',*,*,#1862,.T.);
#2456=ORIENTED_EDGE('',*,*,#1859,.T.);
#2457=ORIENTED_EDGE('',*,*,#1856,.T.);
#2458=ORIENTED_EDGE('',*,*,#1853,.T.);
#2459=ORIENTED_EDGE('',*,*,#1850,.T.);
#2460=ORIENTED_EDGE('',*,*,#1847,.T.);
#2461=ORIENTED_EDGE('',*,*,#1844,.T.);
#2462=ORIENTED_EDGE('',*,*,#1840,.T.);
#2463=ORIENTED_EDGE('',*,*,#1890,.F.);
#2464=ORIENTED_EDGE('',*,*,#1871,.F.);
#2465=ORIENTED_EDGE('',*,*,#1781,.T.);
#2466=ORIENTED_EDGE('',*,*,#1778,.T.);
#2467=ORIENTED_EDGE('',*,*,#1775,.T.);
#2468=ORIENTED_EDGE('',*,*,#1772,.T.);
#2469=ORIENTED_EDGE('',*,*,#1769,.T.);
#2470=ORIENTED_EDGE('',*,*,#1766,.T.);
#2471=ORIENTED_EDGE('',*,*,#1763,.T.);
#2472=ORIENTED_EDGE('',*,*,#1760,.T.);
#2473=ORIENTED_EDGE('',*,*,#1868,.T.);
#2971=CYLINDRICAL_SURFACE('',#3364,0.21);
#3017=ADVANCED_FACE('',(#386),#260,.F.);
#3018=ADVANCED_FACE('',(#387),#261,.F.);
#3019=ADVANCED_FACE('',(#388),#262,.F.);
#3020=ADVANCED_FACE('',(#389),#263,.F.);
#3021=ADVANCED_FACE('',(#390),#264,.F.);
#3022=ADVANCED_FACE('',(#391),#265,.F.);
#3023=ADVANCED_FACE('',(#392),#266,.F.);
#3024=ADVANCED_FACE('',(#393),#267,.F.);
#3025=ADVANCED_FACE('',(#394),#268,.F.);
#3026=ADVANCED_FACE('',(#395),#269,.F.);
#3027=ADVANCED_FACE('',(#396),#270,.F.);
#3028=ADVANCED_FACE('',(#397),#271,.F.);
#3029=ADVANCED_FACE('',(#398),#272,.F.);
#3030=ADVANCED_FACE('',(#399),#273,.F.);
#3031=ADVANCED_FACE('',(#400),#274,.F.);
#3032=ADVANCED_FACE('',(#401),#275,.F.);
#3033=ADVANCED_FACE('',(#402),#276,.F.);
#3034=ADVANCED_FACE('',(#403),#277,.F.);
#3035=ADVANCED_FACE('',(#404),#278,.F.);
#3036=ADVANCED_FACE('',(#405),#279,.F.);
#3037=ADVANCED_FACE('',(#406),#280,.F.);
#3038=ADVANCED_FACE('',(#407),#281,.F.);
#3039=ADVANCED_FACE('',(#408),#282,.F.);
#3040=ADVANCED_FACE('',(#409),#283,.F.);
#3041=ADVANCED_FACE('',(#410),#284,.F.);
#3042=ADVANCED_FACE('',(#411),#285,.F.);
#3043=ADVANCED_FACE('',(#412),#286,.F.);
#3044=ADVANCED_FACE('',(#413),#287,.F.);
#3045=ADVANCED_FACE('',(#414),#288,.F.);
#3046=ADVANCED_FACE('',(#415),#289,.F.);
#3047=ADVANCED_FACE('',(#416),#290,.F.);
#3048=ADVANCED_FACE('',(#417),#291,.F.);
#3049=ADVANCED_FACE('',(#418),#292,.F.);
#3050=ADVANCED_FACE('',(#419),#293,.F.);
#3051=ADVANCED_FACE('',(#420),#294,.F.);
#3052=ADVANCED_FACE('',(#421),#295,.F.);
#3053=ADVANCED_FACE('',(#422),#2971,.F.);
#3054=ADVANCED_FACE('',(#423),#296,.T.);
#3055=ADVANCED_FACE('',(#424),#297,.T.);
#3056=ADVANCED_FACE('',(#425),#298,.T.);
#3057=ADVANCED_FACE('',(#426),#299,.T.);
#3058=ADVANCED_FACE('',(#427),#300,.T.);
#3059=ADVANCED_FACE('',(#428),#301,.T.);
#3060=ADVANCED_FACE('',(#429),#302,.T.);
#3061=ADVANCED_FACE('',(#430),#303,.T.);
#3062=ADVANCED_FACE('',(#431,#222),#304,.T.);
#3063=ADVANCED_FACE('',(#432,#223),#305,.F.);
#3172=CLOSED_SHELL('',(#3017,#3018,#3019,#3020,#3021,#3022,#3023,#3024,
#3025,#3026,#3027,#3028,#3029,#3030,#3031,#3032,#3033,#3034,#3035,#3036,
#3037,#3038,#3039,#3040,#3041,#3042,#3043,#3044,#3045,#3046,#3047,#3048,
#3049,#3050,#3051,#3052,#3053,#3054,#3055,#3056,#3057,#3058,#3059,#3060,
#3061,#3062,#3063));
#3327=AXIS2_PLACEMENT_3D('',#4589,#3676,#3677);
#3328=AXIS2_PLACEMENT_3D('',#4590,#3678,#3679);
#3329=AXIS2_PLACEMENT_3D('',#4599,#3684,#3685);
#3330=AXIS2_PLACEMENT_3D('',#4605,#3689,#3690);
#3331=AXIS2_PLACEMENT_3D('',#4611,#3694,#3695);
#3332=AXIS2_PLACEMENT_3D('',#4617,#3699,#3700);
#3333=AXIS2_PLACEMENT_3D('',#4623,#3704,#3705);
#3334=AXIS2_PLACEMENT_3D('',#4629,#3709,#3710);
#3335=AXIS2_PLACEMENT_3D('',#4635,#3714,#3715);
#3336=AXIS2_PLACEMENT_3D('',#4641,#3719,#3720);
#3337=AXIS2_PLACEMENT_3D('',#4647,#3724,#3725);
#3338=AXIS2_PLACEMENT_3D('',#4656,#3730,#3731);
#3339=AXIS2_PLACEMENT_3D('',#4662,#3735,#3736);
#3340=AXIS2_PLACEMENT_3D('',#4668,#3740,#3741);
#3341=AXIS2_PLACEMENT_3D('',#4674,#3745,#3746);
#3342=AXIS2_PLACEMENT_3D('',#4680,#3750,#3751);
#3343=AXIS2_PLACEMENT_3D('',#4686,#3755,#3756);
#3344=AXIS2_PLACEMENT_3D('',#4692,#3760,#3761);
#3345=AXIS2_PLACEMENT_3D('',#4698,#3765,#3766);
#3346=AXIS2_PLACEMENT_3D('',#4704,#3770,#3771);
#3347=AXIS2_PLACEMENT_3D('',#4713,#3776,#3777);
#3348=AXIS2_PLACEMENT_3D('',#4719,#3781,#3782);
#3349=AXIS2_PLACEMENT_3D('',#4725,#3786,#3787);
#3350=AXIS2_PLACEMENT_3D('',#4731,#3791,#3792);
#3351=AXIS2_PLACEMENT_3D('',#4737,#3796,#3797);
#3352=AXIS2_PLACEMENT_3D('',#4743,#3801,#3802);
#3353=AXIS2_PLACEMENT_3D('',#4749,#3806,#3807);
#3354=AXIS2_PLACEMENT_3D('',#4755,#3811,#3812);
#3355=AXIS2_PLACEMENT_3D('',#4761,#3816,#3817);
#3356=AXIS2_PLACEMENT_3D('',#4770,#3822,#3823);
#3357=AXIS2_PLACEMENT_3D('',#4776,#3827,#3828);
#3358=AXIS2_PLACEMENT_3D('',#4782,#3832,#3833);
#3359=AXIS2_PLACEMENT_3D('',#4788,#3837,#3838);
#3360=AXIS2_PLACEMENT_3D('',#4794,#3842,#3843);
#3361=AXIS2_PLACEMENT_3D('',#4800,#3847,#3848);
#3362=AXIS2_PLACEMENT_3D('',#4806,#3852,#3853);
#3363=AXIS2_PLACEMENT_3D('',#4812,#3857,#3858);
#3364=AXIS2_PLACEMENT_3D('',#4818,#3862,#3863);
#3365=AXIS2_PLACEMENT_3D('',#4820,#3864,#3865);
#3366=AXIS2_PLACEMENT_3D('',#4823,#3867,#3868);
#3367=AXIS2_PLACEMENT_3D('',#4824,#3869,#3870);
#3368=AXIS2_PLACEMENT_3D('',#4830,#3874,#3875);
#3369=AXIS2_PLACEMENT_3D('',#4836,#3879,#3880);
#3370=AXIS2_PLACEMENT_3D('',#4839,#3883,#3884);
#3371=AXIS2_PLACEMENT_3D('',#4845,#3888,#3889);
#3372=AXIS2_PLACEMENT_3D('',#4848,#3892,#3893);
#3373=AXIS2_PLACEMENT_3D('',#4854,#3897,#3898);
#3374=AXIS2_PLACEMENT_3D('',#4857,#3901,#3902);
#3375=AXIS2_PLACEMENT_3D('',#4860,#3905,#3906);
#3376=AXIS2_PLACEMENT_3D('',#4861,#3907,#3908);
#3676=DIRECTION('axis',(0.,0.,1.));
#3677=DIRECTION('refdir',(1.,0.,0.));
#3678=DIRECTION('center_axis',(0.,0.,-1.));
#3679=DIRECTION('ref_axis',(0.,1.,0.));
#3680=DIRECTION('',(0.,1.,0.));
#3681=DIRECTION('',(1.,0.,0.));
#3682=DIRECTION('',(0.,-1.,0.));
#3683=DIRECTION('',(1.,0.,0.));
#3684=DIRECTION('center_axis',(0.,1.,-8.88178419700125E-16));
#3685=DIRECTION('ref_axis',(0.,8.88178419700125E-16,1.));
#3686=DIRECTION('',(0.,8.88178419700125E-16,1.));
#3687=DIRECTION('',(1.,0.,0.));
#3688=DIRECTION('',(0.,-8.88178419700125E-16,-1.));
#3689=DIRECTION('center_axis',(0.,-7.40148683083439E-16,-1.));
#3690=DIRECTION('ref_axis',(0.,1.,-7.40148683083439E-16));
#3691=DIRECTION('',(0.,1.,-7.40148683083439E-16));
#3692=DIRECTION('',(1.,0.,0.));
#3693=DIRECTION('',(0.,-1.,7.40148683083439E-16));
#3694=DIRECTION('center_axis',(0.,-0.707106781186547,-0.707106781186548));
#3695=DIRECTION('ref_axis',(0.,0.707106781186548,-0.707106781186547));
#3696=DIRECTION('',(0.,0.707106781186548,-0.707106781186547));
#3697=DIRECTION('',(1.,0.,0.));
#3698=DIRECTION('',(0.,-0.707106781186548,0.707106781186547));
#3699=DIRECTION('center_axis',(0.,-1.,2.77555756156289E-16));
#3700=DIRECTION('ref_axis',(0.,-2.77555756156289E-16,-1.));
#3701=DIRECTION('',(0.,-2.77555756156289E-16,-1.));
#3702=DIRECTION('',(1.,0.,0.));
#3703=DIRECTION('',(0.,2.77555756156289E-16,1.));
#3704=DIRECTION('center_axis',(0.,-0.707106781186547,0.707106781186548));
#3705=DIRECTION('ref_axis',(0.,-0.707106781186548,-0.707106781186547));
#3706=DIRECTION('',(0.,-0.707106781186548,-0.707106781186547));
#3707=DIRECTION('',(1.,0.,0.));
#3708=DIRECTION('',(0.,0.707106781186548,0.707106781186547));
#3709=DIRECTION('center_axis',(0.,7.40148683083438E-16,1.));
#3710=DIRECTION('ref_axis',(0.,-1.,7.40148683083438E-16));
#3711=DIRECTION('',(0.,-1.,7.40148683083438E-16));
#3712=DIRECTION('',(1.,0.,0.));
#3713=DIRECTION('',(0.,1.,-7.40148683083438E-16));
#3714=DIRECTION('center_axis',(0.,1.,-4.44089209850063E-16));
#3715=DIRECTION('ref_axis',(0.,4.44089209850063E-16,1.));
#3716=DIRECTION('',(0.,4.44089209850063E-16,1.));
#3717=DIRECTION('',(1.,0.,0.));
#3718=DIRECTION('',(0.,-4.44089209850063E-16,-1.));
#3719=DIRECTION('center_axis',(0.,2.41352831440251E-16,1.));
#3720=DIRECTION('ref_axis',(0.,-1.,2.41352831440251E-16));
#3721=DIRECTION('',(0.,-1.,2.41352831440251E-16));
#3722=DIRECTION('',(-1.,0.,0.));
#3723=DIRECTION('',(0.,1.,-2.41352831440251E-16));
#3724=DIRECTION('center_axis',(0.,-1.,2.41352831440251E-16));
#3725=DIRECTION('ref_axis',(0.,-2.41352831440251E-16,-1.));
#3726=DIRECTION('',(0.,-2.41352831440251E-16,-1.));
#3727=DIRECTION('',(1.,0.,0.));
#3728=DIRECTION('',(0.,2.41352831440251E-16,1.));
#3729=DIRECTION('',(1.,0.,0.));
#3730=DIRECTION('center_axis',(0.,0.,-1.));
#3731=DIRECTION('ref_axis',(0.,1.,0.));
#3732=DIRECTION('',(0.,1.,0.));
#3733=DIRECTION('',(1.,0.,0.));
#3734=DIRECTION('',(0.,-1.,0.));
#3735=DIRECTION('center_axis',(0.,-1.,0.));
#3736=DIRECTION('ref_axis',(0.,0.,-1.));
#3737=DIRECTION('',(0.,0.,-1.));
#3738=DIRECTION('',(1.,0.,0.));
#3739=DIRECTION('',(0.,0.,1.));
#3740=DIRECTION('center_axis',(0.,-0.707106781186547,0.707106781186548));
#3741=DIRECTION('ref_axis',(0.,-0.707106781186548,-0.707106781186547));
#3742=DIRECTION('',(0.,-0.707106781186548,-0.707106781186547));
#3743=DIRECTION('',(1.,0.,0.));
#3744=DIRECTION('',(0.,0.707106781186548,0.707106781186547));
#3745=DIRECTION('center_axis',(0.,0.,1.));
#3746=DIRECTION('ref_axis',(0.,-1.,0.));
#3747=DIRECTION('',(0.,-1.,0.));
#3748=DIRECTION('',(1.,0.,0.));
#3749=DIRECTION('',(0.,1.,0.));
#3750=DIRECTION('center_axis',(0.,0.707106781186548,0.707106781186547));
#3751=DIRECTION('ref_axis',(0.,-0.707106781186547,0.707106781186548));
#3752=DIRECTION('',(0.,-0.707106781186547,0.707106781186548));
#3753=DIRECTION('',(1.,0.,0.));
#3754=DIRECTION('',(0.,0.707106781186547,-0.707106781186548));
#3755=DIRECTION('center_axis',(0.,1.,0.));
#3756=DIRECTION('ref_axis',(0.,0.,1.));
#3757=DIRECTION('',(0.,0.,1.));
#3758=DIRECTION('',(1.,0.,0.));
#3759=DIRECTION('',(0.,0.,-1.));
#3760=DIRECTION('center_axis',(0.,0.,-1.));
#3761=DIRECTION('ref_axis',(0.,1.,0.));
#3762=DIRECTION('',(0.,1.,0.));
#3763=DIRECTION('',(1.,0.,0.));
#3764=DIRECTION('',(0.,-1.,0.));
#3765=DIRECTION('center_axis',(0.,1.,-2.41352831440251E-16));
#3766=DIRECTION('ref_axis',(0.,2.41352831440251E-16,1.));
#3767=DIRECTION('',(0.,2.41352831440251E-16,1.));
#3768=DIRECTION('',(-1.,0.,0.));
#3769=DIRECTION('',(0.,-2.41352831440251E-16,-1.));
#3770=DIRECTION('center_axis',(0.,0.,1.));
#3771=DIRECTION('ref_axis',(0.,-1.,0.));
#3772=DIRECTION('',(0.,-1.,0.));
#3773=DIRECTION('',(1.,0.,0.));
#3774=DIRECTION('',(0.,1.,0.));
#3775=DIRECTION('',(1.,0.,0.));
#3776=DIRECTION('center_axis',(0.,-1.,0.));
#3777=DIRECTION('ref_axis',(0.,0.,-1.));
#3778=DIRECTION('',(0.,0.,-1.));
#3779=DIRECTION('',(1.,0.,0.));
#3780=DIRECTION('',(0.,0.,1.));
#3781=DIRECTION('center_axis',(0.,0.,1.));
#3782=DIRECTION('ref_axis',(0.,-1.,0.));
#3783=DIRECTION('',(0.,-1.,0.));
#3784=DIRECTION('',(1.,0.,0.));
#3785=DIRECTION('',(0.,1.,0.));
#3786=DIRECTION('center_axis',(0.,0.707106781186548,0.707106781186548));
#3787=DIRECTION('ref_axis',(0.,-0.707106781186548,0.707106781186548));
#3788=DIRECTION('',(0.,-0.707106781186548,0.707106781186548));
#3789=DIRECTION('',(1.,0.,0.));
#3790=DIRECTION('',(0.,0.707106781186548,-0.707106781186548));
#3791=DIRECTION('center_axis',(0.,1.,0.));
#3792=DIRECTION('ref_axis',(0.,0.,1.));
#3793=DIRECTION('',(0.,0.,1.));
#3794=DIRECTION('',(1.,0.,0.));
#3795=DIRECTION('',(0.,0.,-1.));
#3796=DIRECTION('center_axis',(0.,0.707106781186548,-0.707106781186547));
#3797=DIRECTION('ref_axis',(0.,0.707106781186547,0.707106781186548));
#3798=DIRECTION('',(0.,0.707106781186547,0.707106781186548));
#3799=DIRECTION('',(1.,0.,0.));
#3800=DIRECTION('',(0.,-0.707106781186547,-0.707106781186548));
#3801=DIRECTION('center_axis',(0.,-7.40148683083438E-16,-1.));
#3802=DIRECTION('ref_axis',(0.,1.,-7.40148683083438E-16));
#3803=DIRECTION('',(0.,1.,-7.40148683083438E-16));
#3804=DIRECTION('',(1.,0.,0.));
#3805=DIRECTION('',(0.,-1.,7.40148683083438E-16));
#3806=DIRECTION('center_axis',(0.,-1.,0.));
#3807=DIRECTION('ref_axis',(0.,0.,-1.));
#3808=DIRECTION('',(0.,0.,-1.));
#3809=DIRECTION('',(1.,0.,0.));
#3810=DIRECTION('',(0.,0.,1.));
#3811=DIRECTION('center_axis',(0.,0.,-1.));
#3812=DIRECTION('ref_axis',(0.,1.,0.));
#3813=DIRECTION('',(0.,1.,0.));
#3814=DIRECTION('',(-1.,0.,0.));
#3815=DIRECTION('',(0.,-1.,0.));
#3816=DIRECTION('center_axis',(0.,1.,0.));
#3817=DIRECTION('ref_axis',(0.,0.,1.));
#3818=DIRECTION('',(0.,0.,1.));
#3819=DIRECTION('',(1.,0.,0.));
#3820=DIRECTION('',(0.,0.,-1.));
#3821=DIRECTION('',(1.,0.,0.));
#3822=DIRECTION('center_axis',(0.,0.,1.));
#3823=DIRECTION('ref_axis',(0.,-1.,0.));
#3824=DIRECTION('',(0.,-1.,0.));
#3825=DIRECTION('',(1.,0.,0.));
#3826=DIRECTION('',(0.,1.,0.));
#3827=DIRECTION('center_axis',(0.,1.,0.));
#3828=DIRECTION('ref_axis',(0.,0.,1.));
#3829=DIRECTION('',(0.,0.,1.));
#3830=DIRECTION('',(1.,0.,0.));
#3831=DIRECTION('',(0.,0.,-1.));
#3832=DIRECTION('center_axis',(0.,0.707106781186547,-0.707106781186548));
#3833=DIRECTION('ref_axis',(0.,0.707106781186548,0.707106781186547));
#3834=DIRECTION('',(0.,0.707106781186548,0.707106781186547));
#3835=DIRECTION('',(1.,0.,0.));
#3836=DIRECTION('',(0.,-0.707106781186548,-0.707106781186547));
#3837=DIRECTION('center_axis',(0.,0.,-1.));
#3838=DIRECTION('ref_axis',(0.,1.,0.));
#3839=DIRECTION('',(0.,1.,0.));
#3840=DIRECTION('',(1.,0.,0.));
#3841=DIRECTION('',(0.,-1.,0.));
#3842=DIRECTION('center_axis',(0.,-0.707106781186547,-0.707106781186548));
#3843=DIRECTION('ref_axis',(0.,0.707106781186548,-0.707106781186547));
#3844=DIRECTION('',(0.,0.707106781186548,-0.707106781186547));
#3845=DIRECTION('',(1.,0.,0.));
#3846=DIRECTION('',(0.,-0.707106781186548,0.707106781186547));
#3847=DIRECTION('center_axis',(0.,-1.,0.));
#3848=DIRECTION('ref_axis',(0.,0.,-1.));
#3849=DIRECTION('',(0.,0.,-1.));
#3850=DIRECTION('',(1.,0.,0.));
#3851=DIRECTION('',(0.,0.,1.));
#3852=DIRECTION('center_axis',(0.,0.,1.));
#3853=DIRECTION('ref_axis',(0.,-1.,0.));
#3854=DIRECTION('',(0.,-1.,0.));
#3855=DIRECTION('',(1.,0.,0.));
#3856=DIRECTION('',(0.,1.,0.));
#3857=DIRECTION('center_axis',(0.,-1.,0.));
#3858=DIRECTION('ref_axis',(0.,0.,-1.));
#3859=DIRECTION('',(0.,0.,-1.));
#3860=DIRECTION('',(-1.,0.,0.));
#3861=DIRECTION('',(0.,0.,1.));
#3862=DIRECTION('center_axis',(1.,0.,0.));
#3863=DIRECTION('ref_axis',(0.,0.,-1.));
#3864=DIRECTION('center_axis',(1.,0.,0.));
#3865=DIRECTION('ref_axis',(0.,0.,-1.));
#3866=DIRECTION('',(1.,0.,0.));
#3867=DIRECTION('center_axis',(-1.,0.,0.));
#3868=DIRECTION('ref_axis',(0.,0.,-1.));
#3869=DIRECTION('center_axis',(0.,1.,0.));
#3870=DIRECTION('ref_axis',(0.,0.,1.));
#3871=DIRECTION('',(0.,0.,1.));
#3872=DIRECTION('',(1.,0.,0.));
#3873=DIRECTION('',(0.,0.,1.));
#3874=DIRECTION('center_axis',(0.,1.,0.));
#3875=DIRECTION('ref_axis',(0.,0.,1.));
#3876=DIRECTION('',(0.,0.,1.));
#3877=DIRECTION('',(1.,0.,0.));
#3878=DIRECTION('',(0.,0.,1.));
#3879=DIRECTION('center_axis',(0.,0.,-1.));
#3880=DIRECTION('ref_axis',(0.,1.,0.));
#3881=DIRECTION('',(0.,1.,0.));
#3882=DIRECTION('',(0.,1.,0.));
#3883=DIRECTION('center_axis',(0.,0.,-1.));
#3884=DIRECTION('ref_axis',(0.,1.,0.));
#3885=DIRECTION('',(0.,1.,0.));
#3886=DIRECTION('',(1.,0.,0.));
#3887=DIRECTION('',(0.,1.,0.));
#3888=DIRECTION('center_axis',(0.,-1.,0.));
#3889=DIRECTION('ref_axis',(0.,0.,-1.));
#3890=DIRECTION('',(0.,0.,-1.));
#3891=DIRECTION('',(0.,0.,-1.));
#3892=DIRECTION('center_axis',(0.,-1.,0.));
#3893=DIRECTION('ref_axis',(0.,0.,-1.));
#3894=DIRECTION('',(0.,0.,-1.));
#3895=DIRECTION('',(1.,0.,0.));
#3896=DIRECTION('',(0.,0.,-1.));
#3897=DIRECTION('center_axis',(0.,0.,1.));
#3898=DIRECTION('ref_axis',(0.,-1.,0.));
#3899=DIRECTION('',(0.,-1.,0.));
#3900=DIRECTION('',(0.,-1.,0.));
#3901=DIRECTION('center_axis',(0.,0.,1.));
#3902=DIRECTION('ref_axis',(0.,-1.,0.));
#3903=DIRECTION('',(0.,-1.,0.));
#3904=DIRECTION('',(0.,-1.,0.));
#3905=DIRECTION('center_axis',(1.,0.,0.));
#3906=DIRECTION('ref_axis',(0.,0.,-1.));
#3907=DIRECTION('center_axis',(1.,0.,0.));
#3908=DIRECTION('ref_axis',(0.,0.,-1.));
#4589=CARTESIAN_POINT('',(0.,0.,0.));
#4590=CARTESIAN_POINT('Origin',(-0.1,0.82,-0.3));
#4591=CARTESIAN_POINT('',(0.,0.82,-0.3));
#4592=CARTESIAN_POINT('',(0.,1.,-0.3));
#4593=CARTESIAN_POINT('',(0.,0.41,-0.3));
#4594=CARTESIAN_POINT('',(10.,0.82,-0.3));
#4595=CARTESIAN_POINT('',(-0.1,0.82,-0.3));
#4596=CARTESIAN_POINT('',(10.,1.,-0.3));
#4597=CARTESIAN_POINT('',(10.,0.41,-0.3));
#4598=CARTESIAN_POINT('',(-0.05,1.,-0.3));
#4599=CARTESIAN_POINT('Origin',(-0.1,0.82,-0.55));
#4600=CARTESIAN_POINT('',(0.,0.82,-0.55));
#4601=CARTESIAN_POINT('',(0.,0.82,-0.275));
#4602=CARTESIAN_POINT('',(10.,0.82,-0.55));
#4603=CARTESIAN_POINT('',(-0.1,0.82,-0.55));
#4604=CARTESIAN_POINT('',(10.,0.82,-0.275));
#4605=CARTESIAN_POINT('Origin',(-0.1,0.67,-0.55));
#4606=CARTESIAN_POINT('',(0.,0.67,-0.55));
#4607=CARTESIAN_POINT('',(0.,0.335,-0.55));
#4608=CARTESIAN_POINT('',(10.,0.67,-0.55));
#4609=CARTESIAN_POINT('',(-0.1,0.67,-0.55));
#4610=CARTESIAN_POINT('',(10.,0.335,-0.55));
#4611=CARTESIAN_POINT('Origin',(-0.1,0.42,-0.3));
#4612=CARTESIAN_POINT('',(0.,0.42,-0.3));
#4613=CARTESIAN_POINT('',(0.,0.24,-0.12));
#4614=CARTESIAN_POINT('',(10.,0.42,-0.3));
#4615=CARTESIAN_POINT('',(-0.1,0.42,-0.3));
#4616=CARTESIAN_POINT('',(10.,0.24,-0.12));
#4617=CARTESIAN_POINT('Origin',(-0.1,0.42,0.3));
#4618=CARTESIAN_POINT('',(0.,0.42,0.3));
#4619=CARTESIAN_POINT('',(0.,0.42,0.15));
#4620=CARTESIAN_POINT('',(10.,0.42,0.3));
#4621=CARTESIAN_POINT('',(-0.1,0.42,0.3));
#4622=CARTESIAN_POINT('',(10.,0.42,0.15));
#4623=CARTESIAN_POINT('Origin',(-0.1,0.67,0.55));
#4624=CARTESIAN_POINT('',(0.,0.67,0.55));
#4625=CARTESIAN_POINT('',(6.93889390390723E-18,0.365,0.245));
#4626=CARTESIAN_POINT('',(10.,0.67,0.55));
#4627=CARTESIAN_POINT('',(-0.1,0.67,0.55));
#4628=CARTESIAN_POINT('',(10.,0.365,0.245));
#4629=CARTESIAN_POINT('Origin',(-0.1,0.82,0.55));
#4630=CARTESIAN_POINT('',(0.,0.82,0.55));
#4631=CARTESIAN_POINT('',(0.,0.41,0.55));
#4632=CARTESIAN_POINT('',(10.,0.82,0.55));
#4633=CARTESIAN_POINT('',(-0.1,0.82,0.55));
#4634=CARTESIAN_POINT('',(10.,0.41,0.55));
#4635=CARTESIAN_POINT('Origin',(-0.1,0.82,0.3));
#4636=CARTESIAN_POINT('',(0.,0.82,0.3));
#4637=CARTESIAN_POINT('',(0.,0.82,0.15));
#4638=CARTESIAN_POINT('',(10.,0.82,0.3));
#4639=CARTESIAN_POINT('',(-0.1,0.82,0.3));
#4640=CARTESIAN_POINT('',(10.,0.82,0.15));
#4641=CARTESIAN_POINT('Origin',(-0.1,1.05,0.3));
#4642=CARTESIAN_POINT('',(0.,1.,0.3));
#4643=CARTESIAN_POINT('',(0.,0.525,0.3));
#4644=CARTESIAN_POINT('',(10.,1.,0.3));
#4645=CARTESIAN_POINT('',(-0.05,1.,0.3));
#4646=CARTESIAN_POINT('',(10.,0.525,0.3));
#4647=CARTESIAN_POINT('Origin',(-0.1,-0.3,-0.82));
#4648=CARTESIAN_POINT('',(0.,-0.3,-0.82));
#4649=CARTESIAN_POINT('',(0.,-0.3,-1.));
#4650=CARTESIAN_POINT('',(0.,-0.3,-0.41));
#4651=CARTESIAN_POINT('',(10.,-0.3,-0.82));
#4652=CARTESIAN_POINT('',(-0.1,-0.3,-0.82));
#4653=CARTESIAN_POINT('',(10.,-0.3,-1.));
#4654=CARTESIAN_POINT('',(10.,-0.3,-0.41));
#4655=CARTESIAN_POINT('',(-0.05,-0.3,-1.));
#4656=CARTESIAN_POINT('Origin',(-0.1,-0.55,-0.82));
#4657=CARTESIAN_POINT('',(0.,-0.55,-0.82));
#4658=CARTESIAN_POINT('',(0.,-0.275,-0.82));
#4659=CARTESIAN_POINT('',(10.,-0.55,-0.82));
#4660=CARTESIAN_POINT('',(-0.1,-0.55,-0.82));
#4661=CARTESIAN_POINT('',(10.,-0.275,-0.82));
#4662=CARTESIAN_POINT('Origin',(-0.1,-0.55,-0.67));
#4663=CARTESIAN_POINT('',(0.,-0.55,-0.67));
#4664=CARTESIAN_POINT('',(0.,-0.55,-0.335));
#4665=CARTESIAN_POINT('',(10.,-0.55,-0.67));
#4666=CARTESIAN_POINT('',(-0.1,-0.55,-0.67));
#4667=CARTESIAN_POINT('',(10.,-0.55,-0.335));
#4668=CARTESIAN_POINT('Origin',(-0.1,-0.3,-0.42));
#4669=CARTESIAN_POINT('',(0.,-0.3,-0.42));
#4670=CARTESIAN_POINT('',(0.,-0.12,-0.24));
#4671=CARTESIAN_POINT('',(10.,-0.3,-0.42));
#4672=CARTESIAN_POINT('',(-0.1,-0.3,-0.42));
#4673=CARTESIAN_POINT('',(10.,-0.12,-0.24));
#4674=CARTESIAN_POINT('Origin',(-0.1,0.3,-0.42));
#4675=CARTESIAN_POINT('',(0.,0.3,-0.42));
#4676=CARTESIAN_POINT('',(0.,0.15,-0.42));
#4677=CARTESIAN_POINT('',(10.,0.3,-0.42));
#4678=CARTESIAN_POINT('',(-0.1,0.3,-0.42));
#4679=CARTESIAN_POINT('',(10.,0.15,-0.42));
#4680=CARTESIAN_POINT('Origin',(-0.1,0.55,-0.67));
#4681=CARTESIAN_POINT('',(0.,0.55,-0.67));
#4682=CARTESIAN_POINT('',(0.,0.245,-0.365));
#4683=CARTESIAN_POINT('',(10.,0.55,-0.67));
#4684=CARTESIAN_POINT('',(-0.1,0.55,-0.67));
#4685=CARTESIAN_POINT('',(10.,0.245,-0.365));
#4686=CARTESIAN_POINT('Origin',(-0.1,0.55,-0.82));
#4687=CARTESIAN_POINT('',(0.,0.55,-0.82));
#4688=CARTESIAN_POINT('',(0.,0.55,-0.41));
#4689=CARTESIAN_POINT('',(10.,0.55,-0.82));
#4690=CARTESIAN_POINT('',(-0.1,0.55,-0.82));
#4691=CARTESIAN_POINT('',(10.,0.55,-0.41));
#4692=CARTESIAN_POINT('Origin',(-0.1,0.3,-0.82));
#4693=CARTESIAN_POINT('',(0.,0.3,-0.82));
#4694=CARTESIAN_POINT('',(0.,0.15,-0.82));
#4695=CARTESIAN_POINT('',(10.,0.3,-0.82));
#4696=CARTESIAN_POINT('',(-0.1,0.3,-0.82));
#4697=CARTESIAN_POINT('',(10.,0.15,-0.82));
#4698=CARTESIAN_POINT('Origin',(-0.1,0.3,-1.05));
#4699=CARTESIAN_POINT('',(0.,0.3,-1.));
#4700=CARTESIAN_POINT('',(0.,0.3,-0.525));
#4701=CARTESIAN_POINT('',(10.,0.3,-1.));
#4702=CARTESIAN_POINT('',(-0.05,0.3,-1.));
#4703=CARTESIAN_POINT('',(10.,0.3,-0.525));
#4704=CARTESIAN_POINT('Origin',(-0.1,-0.82,0.3));
#4705=CARTESIAN_POINT('',(0.,-0.82,0.3));
#4706=CARTESIAN_POINT('',(0.,-1.,0.3));
#4707=CARTESIAN_POINT('',(0.,-0.41,0.3));
#4708=CARTESIAN_POINT('',(10.,-0.82,0.3));
#4709=CARTESIAN_POINT('',(-0.1,-0.82,0.3));
#4710=CARTESIAN_POINT('',(10.,-1.,0.3));
#4711=CARTESIAN_POINT('',(10.,-0.41,0.3));
#4712=CARTESIAN_POINT('',(-0.05,-1.,0.3));
#4713=CARTESIAN_POINT('Origin',(-0.1,-0.82,0.55));
#4714=CARTESIAN_POINT('',(0.,-0.82,0.55));
#4715=CARTESIAN_POINT('',(0.,-0.82,0.275));
#4716=CARTESIAN_POINT('',(10.,-0.82,0.55));
#4717=CARTESIAN_POINT('',(-0.1,-0.82,0.55));
#4718=CARTESIAN_POINT('',(10.,-0.82,0.275));
#4719=CARTESIAN_POINT('Origin',(-0.1,-0.67,0.55));
#4720=CARTESIAN_POINT('',(0.,-0.67,0.55));
#4721=CARTESIAN_POINT('',(0.,-0.335,0.55));
#4722=CARTESIAN_POINT('',(10.,-0.67,0.55));
#4723=CARTESIAN_POINT('',(-0.1,-0.67,0.55));
#4724=CARTESIAN_POINT('',(10.,-0.335,0.55));
#4725=CARTESIAN_POINT('Origin',(-0.1,-0.42,0.3));
#4726=CARTESIAN_POINT('',(0.,-0.42,0.3));
#4727=CARTESIAN_POINT('',(-6.93889390390723E-18,-0.24,0.12));
#4728=CARTESIAN_POINT('',(10.,-0.42,0.3));
#4729=CARTESIAN_POINT('',(-0.1,-0.42,0.3));
#4730=CARTESIAN_POINT('',(10.,-0.24,0.12));
#4731=CARTESIAN_POINT('Origin',(-0.1,-0.42,-0.3));
#4732=CARTESIAN_POINT('',(0.,-0.42,-0.3));
#4733=CARTESIAN_POINT('',(0.,-0.42,-0.15));
#4734=CARTESIAN_POINT('',(10.,-0.42,-0.3));
#4735=CARTESIAN_POINT('',(-0.1,-0.42,-0.3));
#4736=CARTESIAN_POINT('',(10.,-0.42,-0.15));
#4737=CARTESIAN_POINT('Origin',(-0.1,-0.67,-0.55));
#4738=CARTESIAN_POINT('',(0.,-0.67,-0.55));
#4739=CARTESIAN_POINT('',(0.,-0.365,-0.245));
#4740=CARTESIAN_POINT('',(10.,-0.67,-0.55));
#4741=CARTESIAN_POINT('',(-0.1,-0.67,-0.55));
#4742=CARTESIAN_POINT('',(10.,-0.365,-0.245));
#4743=CARTESIAN_POINT('Origin',(-0.1,-0.82,-0.55));
#4744=CARTESIAN_POINT('',(0.,-0.82,-0.55));
#4745=CARTESIAN_POINT('',(0.,-0.41,-0.55));
#4746=CARTESIAN_POINT('',(10.,-0.82,-0.55));
#4747=CARTESIAN_POINT('',(-0.1,-0.82,-0.55));
#4748=CARTESIAN_POINT('',(10.,-0.41,-0.55));
#4749=CARTESIAN_POINT('Origin',(-0.1,-0.82,-0.3));
#4750=CARTESIAN_POINT('',(0.,-0.82,-0.3));
#4751=CARTESIAN_POINT('',(0.,-0.82,-0.15));
#4752=CARTESIAN_POINT('',(10.,-0.82,-0.3));
#4753=CARTESIAN_POINT('',(-0.1,-0.82,-0.3));
#4754=CARTESIAN_POINT('',(10.,-0.82,-0.15));
#4755=CARTESIAN_POINT('Origin',(-0.1,-1.05,-0.3));
#4756=CARTESIAN_POINT('',(0.,-1.,-0.3));
#4757=CARTESIAN_POINT('',(0.,-0.525,-0.3));
#4758=CARTESIAN_POINT('',(10.,-1.,-0.3));
#4759=CARTESIAN_POINT('',(-0.05,-1.,-0.3));
#4760=CARTESIAN_POINT('',(10.,-0.525,-0.3));
#4761=CARTESIAN_POINT('Origin',(-0.1,0.3,0.82));
#4762=CARTESIAN_POINT('',(0.,0.3,0.82));
#4763=CARTESIAN_POINT('',(0.,0.3,1.));
#4764=CARTESIAN_POINT('',(0.,0.3,0.41));
#4765=CARTESIAN_POINT('',(10.,0.3,0.82));
#4766=CARTESIAN_POINT('',(-0.1,0.3,0.82));
#4767=CARTESIAN_POINT('',(10.,0.3,1.));
#4768=CARTESIAN_POINT('',(10.,0.3,0.41));
#4769=CARTESIAN_POINT('',(-0.05,0.3,1.));
#4770=CARTESIAN_POINT('Origin',(-0.1,0.55,0.82));
#4771=CARTESIAN_POINT('',(0.,0.55,0.82));
#4772=CARTESIAN_POINT('',(0.,0.275,0.82));
#4773=CARTESIAN_POINT('',(10.,0.55,0.82));
#4774=CARTESIAN_POINT('',(-0.1,0.55,0.82));
#4775=CARTESIAN_POINT('',(10.,0.275,0.82));
#4776=CARTESIAN_POINT('Origin',(-0.1,0.55,0.67));
#4777=CARTESIAN_POINT('',(0.,0.55,0.67));
#4778=CARTESIAN_POINT('',(0.,0.55,0.335));
#4779=CARTESIAN_POINT('',(10.,0.55,0.67));
#4780=CARTESIAN_POINT('',(-0.1,0.55,0.67));
#4781=CARTESIAN_POINT('',(10.,0.55,0.335));
#4782=CARTESIAN_POINT('Origin',(-0.1,0.3,0.42));
#4783=CARTESIAN_POINT('',(0.,0.3,0.42));
#4784=CARTESIAN_POINT('',(6.93889390390723E-18,0.12,0.24));
#4785=CARTESIAN_POINT('',(10.,0.3,0.42));
#4786=CARTESIAN_POINT('',(-0.1,0.3,0.42));
#4787=CARTESIAN_POINT('',(10.,0.12,0.24));
#4788=CARTESIAN_POINT('Origin',(-0.1,-0.3,0.42));
#4789=CARTESIAN_POINT('',(0.,-0.3,0.42));
#4790=CARTESIAN_POINT('',(0.,-0.15,0.42));
#4791=CARTESIAN_POINT('',(10.,-0.3,0.42));
#4792=CARTESIAN_POINT('',(-0.1,-0.3,0.42));
#4793=CARTESIAN_POINT('',(10.,-0.15,0.42));
#4794=CARTESIAN_POINT('Origin',(-0.1,-0.55,0.67));
#4795=CARTESIAN_POINT('',(0.,-0.55,0.67));
#4796=CARTESIAN_POINT('',(6.93889390390723E-18,-0.245,0.365));
#4797=CARTESIAN_POINT('',(10.,-0.55,0.67));
#4798=CARTESIAN_POINT('',(-0.1,-0.55,0.67));
#4799=CARTESIAN_POINT('',(10.,-0.245,0.365));
#4800=CARTESIAN_POINT('Origin',(-0.1,-0.55,0.82));
#4801=CARTESIAN_POINT('',(0.,-0.55,0.82));
#4802=CARTESIAN_POINT('',(0.,-0.55,0.41));
#4803=CARTESIAN_POINT('',(10.,-0.55,0.82));
#4804=CARTESIAN_POINT('',(-0.1,-0.55,0.82));
#4805=CARTESIAN_POINT('',(10.,-0.55,0.41));
#4806=CARTESIAN_POINT('Origin',(-0.1,-0.3,0.82));
#4807=CARTESIAN_POINT('',(0.,-0.3,0.82));
#4808=CARTESIAN_POINT('',(0.,-0.15,0.82));
#4809=CARTESIAN_POINT('',(10.,-0.3,0.82));
#4810=CARTESIAN_POINT('',(-0.1,-0.3,0.82));
#4811=CARTESIAN_POINT('',(10.,-0.15,0.82));
#4812=CARTESIAN_POINT('Origin',(-0.1,-0.3,1.05));
#4813=CARTESIAN_POINT('',(0.,-0.3,1.));
#4814=CARTESIAN_POINT('',(0.,-0.3,0.525));
#4815=CARTESIAN_POINT('',(10.,-0.3,1.));
#4816=CARTESIAN_POINT('',(-0.05,-0.3,1.));
#4817=CARTESIAN_POINT('',(10.,-0.3,0.525));
#4818=CARTESIAN_POINT('Origin',(-0.1,0.,0.));
#4819=CARTESIAN_POINT('',(0.,-2.57175827820944E-17,0.21));
#4820=CARTESIAN_POINT('Origin',(0.,0.,0.));
#4821=CARTESIAN_POINT('',(10.,2.57175827820944E-17,0.21));
#4822=CARTESIAN_POINT('',(-0.1,-2.57175827820944E-17,0.21));
#4823=CARTESIAN_POINT('Origin',(10.,0.,0.));
#4824=CARTESIAN_POINT('Origin',(0.,1.,-1.));
#4825=CARTESIAN_POINT('',(0.,1.,1.));
#4826=CARTESIAN_POINT('',(0.,1.,-1.));
#4827=CARTESIAN_POINT('',(10.,1.,1.));
#4828=CARTESIAN_POINT('',(0.,1.,1.));
#4829=CARTESIAN_POINT('',(10.,1.,-1.));
#4830=CARTESIAN_POINT('Origin',(0.,1.,-1.));
#4831=CARTESIAN_POINT('',(10.,1.,-1.));
#4832=CARTESIAN_POINT('',(10.,1.,-1.));
#4833=CARTESIAN_POINT('',(0.,1.,-1.));
#4834=CARTESIAN_POINT('',(0.,1.,-1.));
#4835=CARTESIAN_POINT('',(0.,1.,-1.));
#4836=CARTESIAN_POINT('Origin',(0.,-1.,-1.));
#4837=CARTESIAN_POINT('',(0.,-1.,-1.));
#4838=CARTESIAN_POINT('',(10.,-1.,-1.));
#4839=CARTESIAN_POINT('Origin',(0.,-1.,-1.));
#4840=CARTESIAN_POINT('',(10.,-1.,-1.));
#4841=CARTESIAN_POINT('',(10.,-1.,-1.));
#4842=CARTESIAN_POINT('',(0.,-1.,-1.));
#4843=CARTESIAN_POINT('',(0.,-1.,-1.));
#4844=CARTESIAN_POINT('',(0.,-1.,-1.));
#4845=CARTESIAN_POINT('Origin',(0.,-1.,1.));
#4846=CARTESIAN_POINT('',(0.,-1.,1.));
#4847=CARTESIAN_POINT('',(10.,-1.,1.));
#4848=CARTESIAN_POINT('Origin',(0.,-1.,1.));
#4849=CARTESIAN_POINT('',(10.,-1.,1.));
#4850=CARTESIAN_POINT('',(10.,-1.,1.));
#4851=CARTESIAN_POINT('',(0.,-1.,1.));
#4852=CARTESIAN_POINT('',(0.,-1.,1.));
#4853=CARTESIAN_POINT('',(0.,-1.,1.));
#4854=CARTESIAN_POINT('Origin',(0.,1.,1.));
#4855=CARTESIAN_POINT('',(0.,1.,1.));
#4856=CARTESIAN_POINT('',(10.,1.,1.));
#4857=CARTESIAN_POINT('Origin',(0.,1.,1.));
#4858=CARTESIAN_POINT('',(10.,1.,1.));
#4859=CARTESIAN_POINT('',(0.,1.,1.));
#4860=CARTESIAN_POINT('Origin',(10.,0.,0.));
#4861=CARTESIAN_POINT('Origin',(0.,0.,0.));
#5462=UNCERTAINTY_MEASURE_WITH_UNIT(LENGTH_MEASURE(0.001),#5493,
'DISTANCE_ACCURACY_VALUE',
'Maximum model space distance between geometric entities at asserted c
onnectivities');
#5475=UNCERTAINTY_MEASURE_WITH_UNIT(LENGTH_MEASURE(0.001),#5493,
'DISTANCE_ACCURACY_VALUE',
'Maximum model space distance between geometric entities at asserted c
onnectivities');
#5479=(
GEOMETRIC_REPRESENTATION_CONTEXT(3)
GLOBAL_UNCERTAINTY_ASSIGNED_CONTEXT((#5462))
GLOBAL_UNIT_ASSIGNED_CONTEXT((#5493,#5495,#5496))
REPRESENTATION_CONTEXT('','3D')
);
#5492=(
GEOMETRIC_REPRESENTATION_CONTEXT(3)
GLOBAL_UNCERTAINTY_ASSIGNED_CONTEXT((#5475))
GLOBAL_UNIT_ASSIGNED_CONTEXT((#5493,#5495,#5496))
REPRESENTATION_CONTEXT('','3D')
);
#5493=(
LENGTH_UNIT()
NAMED_UNIT(*)
SI_UNIT(.CENTI.,.METRE.)
);
#5495=(
NAMED_UNIT(*)
PLANE_ANGLE_UNIT()
SI_UNIT($,.RADIAN.)
);
#5496=(
NAMED_UNIT(*)
SI_UNIT($,.STERADIAN.)
SOLID_ANGLE_UNIT()
);
#5500=SHAPE_DEFINITION_REPRESENTATION(#5516,#5565);
#5516=PRODUCT_DEFINITION_SHAPE('',$,#5582);
#5565=SHAPE_REPRESENTATION('',(#3327),#5479);
#5578=PRODUCT_DEFINITION_CONTEXT('part definition',#5628,'design');
#5582=PRODUCT_DEFINITION('Slotted Extrusion - 20 x 20 x 100 mm',
'Slotted Extrusion - 20 x 20 x 100 mm',#5598,#5578);
#5598=PRODUCT_DEFINITION_FORMATION('',$,#5633);
#5628=APPLICATION_CONTEXT(
'Core Data for Automotive Mechanical Design Process');
#5629=PRODUCT_CONTEXT('part definition',#5628,'mechanical');
#5633=PRODUCT('Slotted Extrusion - 20 x 20 x 100 mm',
'Slotted Extrusion - 20 x 20 x 100 mm',
'Slotted Extrusion - 20 x 20 x 100 mm',(#5629));
#5709=COLOUR_RGB('Off White',0.89,0.88,0.83);
#5710=FILL_AREA_STYLE_COLOUR('',#5709);
#5711=FILL_AREA_STYLE('',(#5710));
#5712=SURFACE_STYLE_FILL_AREA(#5711);
#5713=SURFACE_SIDE_STYLE('',(#5712));
#5714=SURFACE_STYLE_USAGE(.BOTH.,#5713);
#5715=PRESENTATION_STYLE_ASSIGNMENT((#5714));
ENDSEC;
END-ISO-10303-21;
